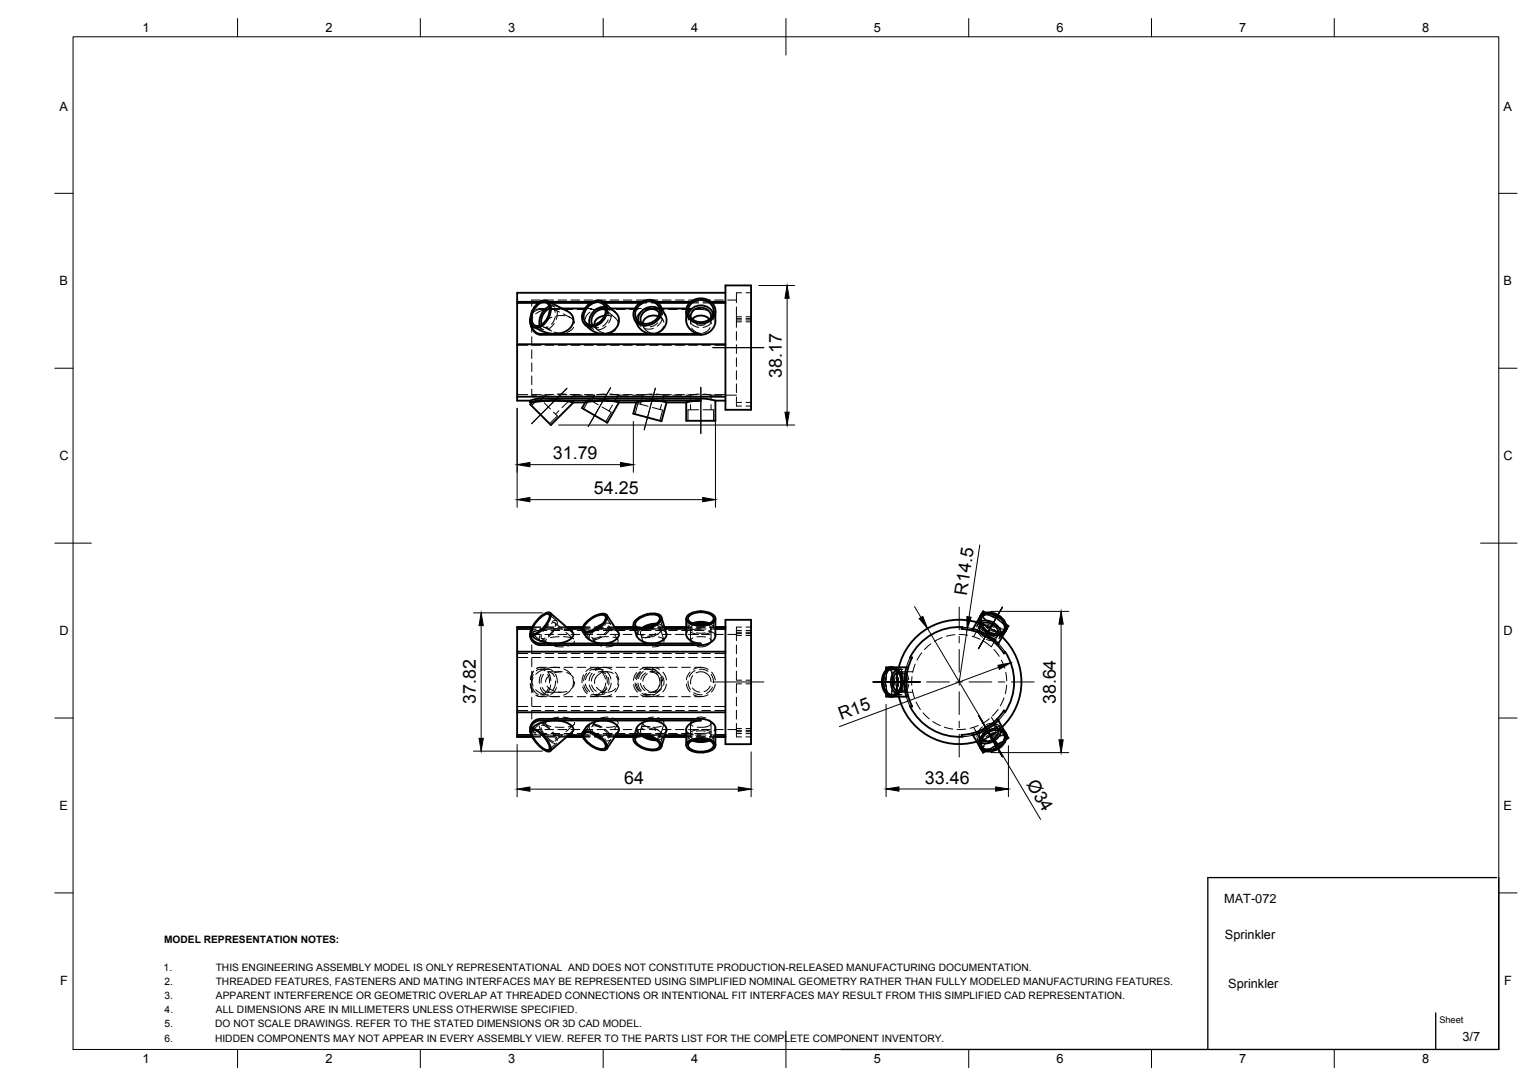
ISO-10303-21;
HEADER;
/* Generated by software containing ST-Developer
 * from STEP Tools, Inc. (www.steptools.com) 
 */

FILE_DESCRIPTION(
/* description */ (''),
/* implementation_level */ '2;1');

FILE_NAME(
/* name */ 'Sprinkler.step',
/* time_stamp */ '2026-10-24T10:30:45-07:00',
/* author */ (''),
/* organization */ (''),
/* preprocessor_version */ 'ST-DEVELOPER v20.2',
/* originating_system */ 'Autodesk Translation Framework v15.15.0.0',
/* authorisation */ '');

FILE_SCHEMA (('AUTOMOTIVE_DESIGN { 1 0 10303 214 3 1 1 }'));
ENDSEC;

DATA;
#10=MECHANICAL_DESIGN_GEOMETRIC_PRESENTATION_REPRESENTATION('',(#77),#5183);
#67=SHAPE_REPRESENTATION_RELATIONSHIP('SRR','None',#5214,#72);
#72=ADVANCED_BREP_SHAPE_REPRESENTATION('',(#82),#5178);
#77=STYLED_ITEM('',(#5247),#82);
#82=MANIFOLD_SOLID_BREP('Sprinkler',#2363);
#87=B_SPLINE_SURFACE_WITH_KNOTS('',3,1,((#4861,#4862),(#4863,#4864),(#4865,
#4866),(#4867,#4868),(#4869,#4870),(#4871,#4872),(#4873,#4874),(#4875,#4876),
(#4877,#4878),(#4879,#4880),(#4881,#4882)),.UNSPECIFIED.,.F.,.F.,.F.,(4,
1,1,1,1,1,1,1,4),(2,2),(3.14159265358979,3.53429173528852,3.92699081698724,
4.31968989868597,4.71238898038469,5.10508806208341,5.49778714378214,5.89048622548086,
6.28318530717959),(0.,0.129347179873149),.UNSPECIFIED.);
#88=B_SPLINE_SURFACE_WITH_KNOTS('',3,1,((#4924,#4925),(#4926,#4927),(#4928,
#4929),(#4930,#4931),(#4932,#4933),(#4934,#4935),(#4936,#4937),(#4938,#4939),
(#4940,#4941),(#4942,#4943),(#4944,#4945)),.UNSPECIFIED.,.F.,.F.,.F.,(4,
1,1,1,1,1,1,1,4),(2,2),(3.14159265358979,3.53429173528851,3.92699081698724,
4.31968989868596,4.71238898038469,5.10508806208341,5.49778714378214,5.89048622548086,
6.28318530717959),(0.,0.129347179873148),.UNSPECIFIED.);
#89=B_SPLINE_SURFACE_WITH_KNOTS('',3,1,((#4987,#4988),(#4989,#4990),(#4991,
#4992),(#4993,#4994),(#4995,#4996),(#4997,#4998),(#4999,#5000),(#5001,#5002),
(#5003,#5004),(#5005,#5006),(#5007,#5008)),.UNSPECIFIED.,.F.,.F.,.F.,(4,
1,1,1,1,1,1,1,4),(2,2),(3.14159265358979,3.53429173528851,3.92699081698723,
4.31968989868596,4.71238898038468,5.10508806208341,5.49778714378213,5.89048622548085,
6.28318530717958),(0.,0.129347179873145),.UNSPECIFIED.);
#90=FACE_BOUND('',#431,.T.);
#91=FACE_BOUND('',#433,.T.);
#92=FACE_BOUND('',#436,.T.);
#93=FACE_BOUND('',#439,.T.);
#94=FACE_BOUND('',#442,.T.);
#95=FACE_BOUND('',#445,.T.);
#96=FACE_BOUND('',#448,.T.);
#97=FACE_BOUND('',#451,.T.);
#98=FACE_BOUND('',#454,.T.);
#99=FACE_BOUND('',#457,.T.);
#100=FACE_BOUND('',#460,.T.);
#101=FACE_BOUND('',#461,.T.);
#102=FACE_BOUND('',#462,.T.);
#103=FACE_BOUND('',#463,.T.);
#104=FACE_BOUND('',#464,.T.);
#105=FACE_BOUND('',#465,.T.);
#106=FACE_BOUND('',#466,.T.);
#107=FACE_BOUND('',#467,.T.);
#108=FACE_BOUND('',#468,.T.);
#109=FACE_BOUND('',#469,.T.);
#110=FACE_BOUND('',#470,.T.);
#111=FACE_BOUND('',#471,.T.);
#112=FACE_BOUND('',#474,.T.);
#113=FACE_BOUND('',#481,.T.);
#114=FACE_BOUND('',#484,.T.);
#115=FACE_BOUND('',#487,.T.);
#116=FACE_BOUND('',#490,.T.);
#117=FACE_BOUND('',#493,.T.);
#118=FACE_BOUND('',#496,.T.);
#119=FACE_BOUND('',#499,.T.);
#120=FACE_BOUND('',#502,.T.);
#121=FACE_BOUND('',#513,.T.);
#122=FACE_BOUND('',#516,.T.);
#123=FACE_BOUND('',#519,.T.);
#124=FACE_BOUND('',#522,.T.);
#125=FACE_BOUND('',#525,.T.);
#126=FACE_BOUND('',#528,.T.);
#127=FACE_BOUND('',#531,.T.);
#128=FACE_BOUND('',#534,.T.);
#129=FACE_BOUND('',#542,.T.);
#130=FACE_BOUND('',#549,.T.);
#131=FACE_BOUND('',#556,.T.);
#144=PLANE('',#2456);
#145=PLANE('',#2461);
#146=PLANE('',#2464);
#147=PLANE('',#2466);
#148=PLANE('',#2470);
#149=PLANE('',#2474);
#150=PLANE('',#2478);
#151=PLANE('',#2482);
#152=PLANE('',#2486);
#153=PLANE('',#2490);
#154=PLANE('',#2494);
#155=PLANE('',#2500);
#156=PLANE('',#2501);
#157=PLANE('',#2509);
#158=PLANE('',#2513);
#159=PLANE('',#2517);
#160=PLANE('',#2521);
#161=PLANE('',#2525);
#162=PLANE('',#2529);
#163=PLANE('',#2533);
#164=PLANE('',#2537);
#165=PLANE('',#2557);
#166=PLANE('',#2560);
#167=PLANE('',#2563);
#168=PLANE('',#2566);
#169=PLANE('',#2569);
#170=PLANE('',#2572);
#171=PLANE('',#2575);
#172=PLANE('',#2578);
#173=PLANE('',#2581);
#174=PLANE('',#2582);
#175=PLANE('',#2583);
#176=PLANE('',#2584);
#177=PLANE('',#2586);
#178=PLANE('',#2587);
#179=PLANE('',#2588);
#180=PLANE('',#2589);
#181=PLANE('',#2591);
#182=PLANE('',#2592);
#183=PLANE('',#2593);
#184=PLANE('',#2594);
#185=PLANE('',#2596);
#186=PLANE('',#2597);
#187=PLANE('',#2598);
#188=PLANE('',#2599);
#189=PLANE('',#2600);
#190=PLANE('',#2601);
#191=PLANE('',#2602);
#192=PLANE('',#2603);
#193=PLANE('',#2604);
#206=B_SPLINE_CURVE_WITH_KNOTS('',3,(#3370,#3371,#3372,#3373,#3374,#3375,
#3376,#3377),.UNSPECIFIED.,.F.,.F.,(4,2,2,4),(0.801601659973552,0.908686694681274,
1.06147652934293,1.21426636400458),.UNSPECIFIED.);
#207=B_SPLINE_CURVE_WITH_KNOTS('',3,(#3379,#3380,#3381,#3382,#3383,#3384,
#3385,#3386,#3387,#3388,#3389,#3390,#3391,#3392),.UNSPECIFIED.,.F.,.F.,
(4,2,2,2,2,2,4),(0.,0.152789834661652,0.305579669323305,0.456356425662796,
0.607133182002287,0.757909938341781,0.801601659973552),.UNSPECIFIED.);
#208=B_SPLINE_CURVE_WITH_KNOTS('',3,(#3396,#3397,#3398,#3399,#3400,#3401,
#3402,#3403,#3404,#3405,#3406,#3407,#3408,#3409,#3410,#3411),
 .UNSPECIFIED.,.F.,.F.,(4,2,2,2,2,2,2,4),(1.41258149283994,1.51470567835646,
1.66615965590029,1.81761363344413,1.96906761098797,2.12052158853181,2.27200321656199,
2.42348484459217),.UNSPECIFIED.);
#209=B_SPLINE_CURVE_WITH_KNOTS('',3,(#3412,#3413,#3414,#3415,#3416,#3417),
 .UNSPECIFIED.,.F.,.F.,(4,2,4),(1.21174242229609,1.36322405032627,1.41258149283994),
 .UNSPECIFIED.);
#210=B_SPLINE_CURVE_WITH_KNOTS('',3,(#3422,#3423,#3424,#3425,#3426,#3427,
#3428,#3429),.UNSPECIFIED.,.F.,.F.,(4,2,2,4),(0.810459053731311,0.931112082660273,
1.09792489409666,1.26473770553305),.UNSPECIFIED.);
#211=B_SPLINE_CURVE_WITH_KNOTS('',3,(#3431,#3432,#3433,#3434,#3435,#3436,
#3437,#3438,#3439,#3440,#3441,#3442,#3443,#3444),.UNSPECIFIED.,.F.,.F.,
(4,2,2,2,2,2,4),(0.,0.166812811436392,0.333625622872784,0.482997237819655,
0.632368852766526,0.781740467713401,0.810459053731311),.UNSPECIFIED.);
#212=B_SPLINE_CURVE_WITH_KNOTS('',3,(#3446,#3447,#3448,#3449,#3450,#3451,
#3452,#3453,#3454,#3455,#3456,#3457,#3458,#3459,#3460,#3461,#3462,#3463),
 .UNSPECIFIED.,.F.,.F.,(4,2,2,2,2,2,2,2,4),(1.21426636400458,1.37281902636882,
1.53137168873306,1.68587949128402,1.84038729383497,1.99489509638593,2.14940289893689,
2.30795556130114,2.46650822366539),.UNSPECIFIED.);
#213=B_SPLINE_CURVE_WITH_KNOTS('',3,(#3468,#3469,#3470,#3471,#3472,#3473,
#3474,#3475,#3476,#3477),.UNSPECIFIED.,.F.,.F.,(4,2,2,2,4),(0.84921255840186,
0.855460999411689,1.0133776521287,1.20423317275903,1.39508869338936),
 .UNSPECIFIED.);
#214=B_SPLINE_CURVE_WITH_KNOTS('',3,(#3479,#3480,#3481,#3482,#3483,#3484,
#3485,#3486,#3487,#3488,#3489,#3490),.UNSPECIFIED.,.F.,.F.,(4,2,2,2,2,4),
(0.,0.19085552063033,0.38171104126066,0.539627693977667,0.697544346694674,
0.84921255840186),.UNSPECIFIED.);
#215=B_SPLINE_CURVE_WITH_KNOTS('',3,(#3492,#3493,#3494,#3495,#3496,#3497,
#3498,#3499,#3500,#3501,#3502,#3503,#3504,#3505,#3506,#3507,#3508,#3509),
 .UNSPECIFIED.,.F.,.F.,(4,2,2,2,2,2,2,2,4),(1.26473770553305,1.44115993597425,
1.61758216641546,1.77878219205947,1.93998221770349,2.10118224334752,2.26238226899155,
2.43880449943275,2.61522672987395),.UNSPECIFIED.);
#216=B_SPLINE_CURVE_WITH_KNOTS('',3,(#3513,#3514,#3515,#3516,#3517,#3518,
#3519,#3520,#3521,#3522,#3523,#3524,#3525,#3526,#3527,#3528,#3529,#3530,
#3531,#3532,#3533,#3534),.UNSPECIFIED.,.F.,.F.,(4,2,2,2,2,2,2,2,2,2,4),
(1.39508869338936,1.63068735474474,1.86628601610013,2.01895939966093,2.09529609144134,
2.17163278322174,2.24796947500215,2.32430616678255,2.47697955034337,2.71257821169876,
2.94817687305416),.UNSPECIFIED.);
#217=B_SPLINE_CURVE_WITH_KNOTS('',3,(#3537,#3538,#3539,#3540,#3541,#3542,
#3543,#3544,#3545,#3546,#3547,#3548,#3549,#3550,#3551,#3552,#3553,#3554,
#3555,#3556,#3557,#3558,#3559,#3560,#3561,#3562),.UNSPECIFIED.,.F.,.F.,
(4,2,2,2,2,2,2,2,2,2,2,2,4),(0.,0.0444658256706816,0.109825747467382,0.210987273969983,
0.363115011869221,0.476603266918211,0.543343022865724,0.610052308554092,
0.7232875236507,0.87579543247345,0.97697424211648,1.04237097445545,1.08685368328188),
 .UNSPECIFIED.);
#218=B_SPLINE_CURVE_WITH_KNOTS('',3,(#3577,#3578,#3579,#3580,#3581,#3582,
#3583,#3584),.UNSPECIFIED.,.F.,.F.,(4,2,2,4),(0.801601659973551,0.908686694681269,
1.06147652934292,1.21426636400457),.UNSPECIFIED.);
#219=B_SPLINE_CURVE_WITH_KNOTS('',3,(#3586,#3587,#3588,#3589,#3590,#3591,
#3592,#3593,#3594,#3595,#3596,#3597,#3598,#3599),.UNSPECIFIED.,.F.,.F.,
(4,2,2,2,2,2,4),(0.,0.152789834661651,0.305579669323302,0.456356425662796,
0.607133182002289,0.757909938341779,0.801601659973551),.UNSPECIFIED.);
#220=B_SPLINE_CURVE_WITH_KNOTS('',3,(#3603,#3604,#3605,#3606,#3607,#3608,
#3609,#3610,#3611,#3612,#3613,#3614,#3615,#3616,#3617,#3618),
 .UNSPECIFIED.,.F.,.F.,(4,2,2,2,2,2,2,4),(1.41258149283993,1.51470567835645,
1.66615965590029,1.81761363344413,1.96906761098797,2.1205215885318,2.27200321656199,
2.42348484459217),.UNSPECIFIED.);
#221=B_SPLINE_CURVE_WITH_KNOTS('',3,(#3619,#3620,#3621,#3622,#3623,#3624),
 .UNSPECIFIED.,.F.,.F.,(4,2,4),(1.21174242229609,1.36322405032627,1.41258149283993),
 .UNSPECIFIED.);
#222=B_SPLINE_CURVE_WITH_KNOTS('',3,(#3629,#3630,#3631,#3632,#3633,#3634,
#3635,#3636),.UNSPECIFIED.,.F.,.F.,(4,2,2,4),(0.810459053731318,0.931112082660271,
1.09792489409666,1.26473770553306),.UNSPECIFIED.);
#223=B_SPLINE_CURVE_WITH_KNOTS('',3,(#3638,#3639,#3640,#3641,#3642,#3643,
#3644,#3645,#3646,#3647,#3648,#3649,#3650,#3651),.UNSPECIFIED.,.F.,.F.,
(4,2,2,2,2,2,4),(0.,0.166812811436393,0.333625622872785,0.482997237819654,
0.632368852766523,0.781740467713397,0.810459053731318),.UNSPECIFIED.);
#224=B_SPLINE_CURVE_WITH_KNOTS('',3,(#3653,#3654,#3655,#3656,#3657,#3658,
#3659,#3660,#3661,#3662,#3663,#3664,#3665,#3666,#3667,#3668,#3669,#3670),
 .UNSPECIFIED.,.F.,.F.,(4,2,2,2,2,2,2,2,4),(1.21426636400457,1.37281902636881,
1.53137168873306,1.68587949128401,1.84038729383497,1.99489509638593,2.14940289893689,
2.30795556130114,2.46650822366538),.UNSPECIFIED.);
#225=B_SPLINE_CURVE_WITH_KNOTS('',3,(#3675,#3676,#3677,#3678,#3679,#3680,
#3681,#3682),.UNSPECIFIED.,.F.,.F.,(4,2,2,4),(0.848478832255458,0.991796836691898,
1.19347267089766,1.39514850510343),.UNSPECIFIED.);
#226=B_SPLINE_CURVE_WITH_KNOTS('',3,(#3684,#3685,#3686,#3687,#3688,#3689,
#3690,#3691,#3692,#3693,#3694,#3695,#3696,#3697),.UNSPECIFIED.,.F.,.F.,
(4,2,2,2,2,2,4),(0.,0.201675834205757,0.403351668411514,0.550462960481608,
0.697574252551703,0.8446855446218,0.848478832255458),.UNSPECIFIED.);
#227=B_SPLINE_CURVE_WITH_KNOTS('',3,(#3699,#3700,#3701,#3702,#3703,#3704,
#3705,#3706,#3707,#3708,#3709,#3710,#3711,#3712,#3713,#3714,#3715,#3716),
 .UNSPECIFIED.,.F.,.F.,(4,2,2,2,2,2,2,2,4),(1.26473770553306,1.44115993597426,
1.61758216641546,1.77878219205948,1.93998221770349,2.10118224334752,2.26238226899154,
2.43880449943275,2.61522672987395),.UNSPECIFIED.);
#228=B_SPLINE_CURVE_WITH_KNOTS('',3,(#3720,#3721,#3722,#3723,#3724,#3725,
#3726,#3727,#3728,#3729,#3730,#3731,#3732,#3733,#3734,#3735,#3736,#3737,
#3738,#3739,#3740,#3741),.UNSPECIFIED.,.F.,.F.,(4,2,2,2,2,2,2,2,2,2,4),
(1.39514850510343,1.60860320712188,1.82205790914033,1.99791237111712,2.08583960210551,
2.17376683309391,2.26169406408231,2.34962129507071,2.5254757570475,2.73893045906596,
2.95238516108442),.UNSPECIFIED.);
#229=B_SPLINE_CURVE_WITH_KNOTS('',3,(#3744,#3745,#3746,#3747,#3748,#3749,
#3750,#3751,#3752,#3753,#3754,#3755,#3756,#3757,#3758,#3759,#3760,#3761,
#3762,#3763,#3764,#3765,#3766,#3767,#3768,#3769),.UNSPECIFIED.,.F.,.F.,
(4,2,2,2,2,2,2,2,2,2,2,2,4),(0.,0.0444658256707017,0.109825747467453,0.210987273970143,
0.363115011869592,0.4766032669186,0.543343022866364,0.610052308555067,0.723287523653244,
0.875795432478097,0.97697424212264,1.04237097446268,1.08685368328966),
 .UNSPECIFIED.);
#230=B_SPLINE_CURVE_WITH_KNOTS('',3,(#3775,#3776,#3777,#3778,#3779,#3780,
#3781,#3782),.UNSPECIFIED.,.F.,.F.,(4,2,2,4),(0.80160165997355,0.908686694681275,
1.06147652934293,1.21426636400458),.UNSPECIFIED.);
#231=B_SPLINE_CURVE_WITH_KNOTS('',3,(#3784,#3785,#3786,#3787,#3788,#3789,
#3790,#3791,#3792,#3793,#3794,#3795,#3796,#3797),.UNSPECIFIED.,.F.,.F.,
(4,2,2,2,2,2,4),(0.,0.152789834661653,0.305579669323305,0.456356425662799,
0.607133182002292,0.757909938341784,0.80160165997355),.UNSPECIFIED.);
#232=B_SPLINE_CURVE_WITH_KNOTS('',3,(#3801,#3802,#3803,#3804,#3805,#3806,
#3807,#3808,#3809,#3810,#3811,#3812,#3813,#3814,#3815,#3816),
 .UNSPECIFIED.,.F.,.F.,(4,2,2,2,2,2,2,4),(1.41258149283993,1.51470567835645,
1.66615965590029,1.81761363344413,1.96906761098797,2.12052158853181,2.27200321656199,
2.42348484459217),.UNSPECIFIED.);
#233=B_SPLINE_CURVE_WITH_KNOTS('',3,(#3817,#3818,#3819,#3820,#3821,#3822),
 .UNSPECIFIED.,.F.,.F.,(4,2,4),(1.21174242229609,1.36322405032627,1.41258149283993),
 .UNSPECIFIED.);
#234=B_SPLINE_CURVE_WITH_KNOTS('',3,(#3827,#3828,#3829,#3830,#3831,#3832,
#3833,#3834),.UNSPECIFIED.,.F.,.F.,(4,2,2,4),(0.810451797988797,0.931104826917751,
1.09791763835414,1.26473044979053),.UNSPECIFIED.);
#235=B_SPLINE_CURVE_WITH_KNOTS('',3,(#3836,#3837,#3838,#3839,#3840,#3841,
#3842,#3843,#3844,#3845,#3846,#3847,#3848,#3849),.UNSPECIFIED.,.F.,.F.,
(4,2,2,2,2,2,4),(0.,0.163827053405726,0.327654106811452,0.48000785191773,
0.632361597024009,0.781733211970881,0.810451797988797),.UNSPECIFIED.);
#236=B_SPLINE_CURVE_WITH_KNOTS('',3,(#3851,#3852,#3853,#3854,#3855,#3856,
#3857,#3858,#3859,#3860,#3861,#3862,#3863,#3864,#3865,#3866,#3867,#3868),
 .UNSPECIFIED.,.F.,.F.,(4,2,2,2,2,2,2,2,4),(1.21426636400458,1.37281902636882,
1.53137168873306,1.68587949128402,1.84038729383497,1.99489509638594,2.1494028989369,
2.30795556130114,2.46650822366539),.UNSPECIFIED.);
#237=B_SPLINE_CURVE_WITH_KNOTS('',3,(#3873,#3874,#3875,#3876,#3877,#3878,
#3879,#3880,#3881,#3882),.UNSPECIFIED.,.F.,.F.,(4,2,2,2,4),(0.849212558401863,
0.855460999411694,1.01337765212871,1.20423317275904,1.39508869338936),
 .UNSPECIFIED.);
#238=B_SPLINE_CURVE_WITH_KNOTS('',3,(#3884,#3885,#3886,#3887,#3888,#3889,
#3890,#3891,#3892,#3893,#3894,#3895),.UNSPECIFIED.,.F.,.F.,(4,2,2,2,2,4),
(0.,0.190855520630331,0.381711041260663,0.539627693977671,0.697544346694678,
0.849212558401863),.UNSPECIFIED.);
#239=B_SPLINE_CURVE_WITH_KNOTS('',3,(#3897,#3898,#3899,#3900,#3901,#3902,
#3903,#3904,#3905,#3906,#3907,#3908,#3909,#3910,#3911,#3912,#3913,#3914),
 .UNSPECIFIED.,.F.,.F.,(4,2,2,2,2,2,2,2,4),(1.26473044979053,1.45047293867533,
1.63621542756013,1.78793284105988,1.93965025455964,2.0913676680594,2.24308508155916,
2.42882757044396,2.61457005932877),.UNSPECIFIED.);
#240=B_SPLINE_CURVE_WITH_KNOTS('',3,(#3918,#3919,#3920,#3921,#3922,#3923,
#3924,#3925,#3926,#3927,#3928,#3929,#3930,#3931,#3932,#3933,#3934,#3935,
#3936,#3937,#3938,#3939),.UNSPECIFIED.,.F.,.F.,(4,2,2,2,2,2,2,2,2,2,4),
(1.39508869338936,1.63068735474475,1.86628601610013,2.01895939966094,2.09529609144135,
2.17163278322175,2.24796947500216,2.32430616678257,2.47697955034339,2.71257821169878,
2.94817687305417),.UNSPECIFIED.);
#241=B_SPLINE_CURVE_WITH_KNOTS('',3,(#3942,#3943,#3944,#3945,#3946,#3947,
#3948,#3949,#3950,#3951,#3952,#3953,#3954,#3955,#3956,#3957,#3958,#3959,
#3960,#3961,#3962,#3963,#3964,#3965,#3966,#3967),.UNSPECIFIED.,.F.,.F.,
(4,2,2,2,2,2,2,2,2,2,2,2,4),(0.,0.0444658256707104,0.109825747467599,0.210987273970278,
0.3631150118696,0.476603266918339,0.54334302286555,0.610052308553677,0.723287523650531,
0.875795432473984,0.97697424211741,1.0423709744566,1.08685368328313),
 .UNSPECIFIED.);
#242=B_SPLINE_CURVE_WITH_KNOTS('',3,(#4068,#4069,#4070,#4071,#4072,#4073,
#4074,#4075,#4076,#4077,#4078,#4079,#4080,#4081,#4082,#4083,#4084,#4085),
 .UNSPECIFIED.,.F.,.F.,(4,2,2,2,2,2,2,2,4),(-2.42440986895006,-2.27286833474306,
-2.12132680053607,-1.9698171011243,-1.81830740171254,-1.66679770230078,
-1.51528800288901,-1.36374646868202,-1.21220493447502),.UNSPECIFIED.);
#243=B_SPLINE_CURVE_WITH_KNOTS('',3,(#4135,#4136,#4137,#4138,#4139,#4140,
#4141,#4142,#4143,#4144,#4145,#4146,#4147,#4148,#4149,#4150,#4151,#4152,
#4153,#4154,#4155),.UNSPECIFIED.,.F.,.F.,(4,2,2,2,3,2,2,2,2,4),(1.63431795680218,
1.63484051213071,1.74655213492763,1.90358589296679,2.06061965100595,2.19559646985844,
2.33057328871092,2.44200600177385,2.55343871483678,2.66004451397958),
 .UNSPECIFIED.);
#244=B_SPLINE_CURVE_WITH_KNOTS('',3,(#4156,#4157,#4158,#4159,#4160,#4161,
#4162,#4163,#4164,#4165,#4166,#4167,#4168,#4169,#4170,#4171,#4172,#4173,
#4174,#4175,#4176,#4177,#4178,#4179),.UNSPECIFIED.,.F.,.F.,(4,2,2,2,2,2,
2,2,2,2,2,4),(2.66004451397958,2.66487142789972,2.77630414096266,2.91128095981515,
3.04625777866764,3.20329153670679,3.36032529474595,3.47203691754285,3.5278927289413,
3.58374854033975,3.63960435173821,3.69493760780813),.UNSPECIFIED.);
#245=B_SPLINE_CURVE_WITH_KNOTS('',3,(#4182,#4183,#4184,#4185,#4186,#4187,
#4188,#4189,#4190,#4191,#4192,#4193,#4194,#4195,#4196,#4197,#4198,#4199,
#4200,#4201,#4202,#4203,#4204),.UNSPECIFIED.,.F.,.F.,(4,2,2,2,3,2,2,2,2,
2,4),(1.63645246149242,1.6458071028209,1.76735674157733,1.91500283165642,
2.06264892173552,2.21065304350676,2.35865716527801,2.45711954510512,2.55558192493224,
2.65404430475936,2.66124396153498),.UNSPECIFIED.);
#246=B_SPLINE_CURVE_WITH_KNOTS('',3,(#4205,#4206,#4207,#4208,#4209,#4210,
#4211,#4212,#4213,#4214,#4215,#4216,#4217,#4218,#4219,#4220,#4221,#4222,
#4223,#4224,#4225,#4226),.UNSPECIFIED.,.F.,.F.,(4,2,2,2,2,2,2,2,2,2,4),
(2.66124396153498,2.75250668458648,2.90051080635773,3.04851492812899,3.19616101820807,
3.34380710828715,3.46535674704357,3.52613156642178,3.58690638579999,3.64768120517821,
3.69910138322794),.UNSPECIFIED.);
#247=B_SPLINE_CURVE_WITH_KNOTS('',3,(#4229,#4230,#4231,#4232,#4233,#4234,
#4235,#4236,#4237,#4238,#4239,#4240,#4241,#4242,#4243,#4244,#4245,#4246,
#4247,#4248,#4249),.UNSPECIFIED.,.F.,.F.,(4,2,2,3,2,2,2,2,2,4),(1.48658026968319,
1.57668032617585,1.70181043495793,1.82694054374001,1.94229840394621,2.0576562641524,
2.16466765320846,2.27167904226452,2.37869043132058,2.39673280800115),
 .UNSPECIFIED.);
#248=B_SPLINE_CURVE_WITH_KNOTS('',3,(#4250,#4251,#4252,#4253,#4254,#4255,
#4256,#4257,#4258,#4259,#4260,#4261,#4262,#4263,#4264,#4265,#4266,#4267,
#4268,#4269),.UNSPECIFIED.,.F.,.F.,(4,2,2,2,2,2,2,2,2,4),(2.39673280800115,
2.48570182037664,2.60105968058284,2.71641754078903,2.84154764957111,2.96667775835319,
3.07591353624385,3.18514931413451,3.29438509202518,3.3135208134232),
 .UNSPECIFIED.);
#249=B_SPLINE_CURVE_WITH_KNOTS('',3,(#4272,#4273,#4274,#4275,#4276,#4277,
#4278,#4279,#4280,#4281,#4282,#4283,#4284,#4285,#4286,#4287,#4288,#4289,
#4290,#4291,#4292),.UNSPECIFIED.,.F.,.F.,(4,2,2,3,2,2,2,2,2,4),(1.48667142164751,
1.57677147814025,1.70190158692234,1.82703169570442,1.94802136665288,2.06901103760135,
2.17041340390623,2.27181577021112,2.37321813651602,2.39644556681379),
 .UNSPECIFIED.);
#250=B_SPLINE_CURVE_WITH_KNOTS('',3,(#4293,#4294,#4295,#4296,#4297,#4298,
#4299,#4300,#4301,#4302,#4303,#4304,#4305,#4306,#4307,#4308,#4309,#4310,
#4311,#4312),.UNSPECIFIED.,.F.,.F.,(4,2,2,2,2,2,2,2,2,4),(2.39644556681379,
2.47462050282091,2.59561017376938,2.71659984471785,2.84172995349992,2.966860062282,
3.07609584017266,3.18533161806333,3.294567395954,3.31370311735193),
 .UNSPECIFIED.);
#251=B_SPLINE_CURVE_WITH_KNOTS('',3,(#4315,#4316,#4317,#4318,#4319,#4320,
#4321,#4322,#4323,#4324,#4325,#4326,#4327,#4328,#4329,#4330,#4331,#4332,
#4333,#4334,#4335),.UNSPECIFIED.,.F.,.F.,(4,2,2,3,2,2,2,2,2,4),(1.42510602309759,
1.50257240162674,1.61295870334865,1.72334500507057,1.83225417045197,1.94116333583337,
2.04500754168813,2.1488517475429,2.25269595339766,2.2848744256183),
 .UNSPECIFIED.);
#252=B_SPLINE_CURVE_WITH_KNOTS('',3,(#4336,#4337,#4338,#4339,#4340,#4341,
#4342,#4343,#4344,#4345,#4346,#4347,#4348,#4349,#4350,#4351,#4352,#4353,
#4354,#4355),.UNSPECIFIED.,.F.,.F.,(4,2,2,2,2,2,2,2,2,4),(2.2848744256183,
2.35654015925242,2.46544932463382,2.57435849001523,2.68474479173714,2.79513109345905,
2.90282767176861,3.01052425007817,3.11822082838774,3.14845102816816),
 .UNSPECIFIED.);
#253=B_SPLINE_CURVE_WITH_KNOTS('',3,(#4358,#4359,#4360,#4361,#4362,#4363,
#4364,#4365,#4366,#4367,#4368,#4369,#4370,#4371,#4372,#4373,#4374,#4375,
#4376,#4377,#4378),.UNSPECIFIED.,.F.,.F.,(4,2,2,3,2,2,2,2,2,4),(1.42506934481542,
1.50220099251643,1.61276096598296,1.72332093944948,1.83050112648501,1.93768131352053,
2.04324956210919,2.14881781069785,2.25438605928651,2.28497277338716),
 .UNSPECIFIED.);
#254=B_SPLINE_CURVE_WITH_KNOTS('',3,(#4379,#4380,#4381,#4382,#4383,#4384,
#4385,#4386,#4387,#4388,#4389,#4390,#4391,#4392,#4393,#4394,#4395,#4396,
#4397,#4398),.UNSPECIFIED.,.F.,.F.,(4,2,2,2,2,2,2,2,2,4),(2.28497277338716,
2.35995430787517,2.46713449491069,2.57431468194622,2.68487465541274,2.79543462887926,
2.90295645465092,3.01047828042258,3.11800010619425,3.1483902842649),
 .UNSPECIFIED.);
#255=B_SPLINE_CURVE_WITH_KNOTS('',3,(#4401,#4402,#4403,#4404,#4405,#4406,
#4407,#4408,#4409,#4410,#4411,#4412,#4413,#4414,#4415,#4416,#4417,#4418,
#4419,#4420),.UNSPECIFIED.,.F.,.F.,(4,2,2,2,2,2,2,2,2,4),(0.140389663816896,
0.211667950083815,0.317493899242379,0.423319848400943,0.529145797559505,
0.634971746718067,0.740805721759974,0.846639696801881,0.952473671843789,
0.987029360618753),.UNSPECIFIED.);
#256=B_SPLINE_CURVE_WITH_KNOTS('',3,(#4421,#4422,#4423,#4424,#4425,#4426,
#4427,#4428,#4429,#4430,#4431,#4432,#4433,#4434,#4435,#4436,#4437,#4438,
#4439,#4440,#4441),.UNSPECIFIED.,.F.,.F.,(4,2,2,2,2,2,2,3,2,4),(0.987029360618753,
1.0583076468857,1.16413359604426,1.26995954520282,1.37578549436138,1.48161144351995,
1.58744541856186,1.69327939360377,1.79911336864567,1.83366905742066),
 .UNSPECIFIED.);
#257=B_SPLINE_CURVE_WITH_KNOTS('',3,(#4444,#4445,#4446,#4447,#4448,#4449,
#4450,#4451,#4452,#4453,#4454,#4455,#4456,#4457,#4458,#4459,#4460,#4461,
#4462,#4463),.UNSPECIFIED.,.F.,.F.,(4,2,2,2,2,2,2,2,2,4),(0.14038966381692,
0.211667950083817,0.317493899242381,0.423319848400946,0.529145797559508,
0.634971746718069,0.740805721759977,0.846639696801884,0.952473671843792,
0.987029360618756),.UNSPECIFIED.);
#258=B_SPLINE_CURVE_WITH_KNOTS('',3,(#4464,#4465,#4466,#4467,#4468,#4469,
#4470,#4471,#4472,#4473,#4474,#4475,#4476,#4477,#4478,#4479,#4480,#4481,
#4482,#4483,#4484),.UNSPECIFIED.,.F.,.F.,(4,2,2,2,2,2,2,3,2,4),(0.987029360618756,
1.0583076468857,1.16413359604426,1.26995954520282,1.37578549436139,1.48161144351995,
1.58744541856186,1.69327939360377,1.79911336864568,1.83366905742069),
 .UNSPECIFIED.);
#259=B_SPLINE_CURVE_WITH_KNOTS('',3,(#4487,#4488,#4489,#4490,#4491,#4492,
#4493,#4494,#4495,#4496,#4497,#4498,#4499,#4500,#4501,#4502,#4503,#4504,
#4505,#4506,#4507),.UNSPECIFIED.,.F.,.F.,(4,2,2,2,3,2,2,2,2,4),(1.63431795680214,
1.63484051213073,1.74655213492764,1.90358589296679,2.06061965100595,2.19559646985844,
2.33057328871092,2.44200600177386,2.5534387148368,2.66004451397959),
 .UNSPECIFIED.);
#260=B_SPLINE_CURVE_WITH_KNOTS('',3,(#4508,#4509,#4510,#4511,#4512,#4513,
#4514,#4515,#4516,#4517,#4518,#4519,#4520,#4521,#4522,#4523,#4524,#4525,
#4526,#4527,#4528,#4529,#4530,#4531),.UNSPECIFIED.,.F.,.F.,(4,2,2,2,2,2,
2,2,2,2,2,4),(2.66004451397959,2.66487142789973,2.77630414096267,2.91128095981515,
3.04625777866764,3.2032915367068,3.36032529474595,3.47203691754286,3.52789272894132,
3.58374854033977,3.63960435173823,3.69493760780809),.UNSPECIFIED.);
#261=B_SPLINE_CURVE_WITH_KNOTS('',3,(#4534,#4535,#4536,#4537,#4538,#4539,
#4540,#4541,#4542,#4543,#4544,#4545,#4546,#4547,#4548,#4549,#4550,#4551,
#4552,#4553,#4554),.UNSPECIFIED.,.F.,.F.,(4,2,2,3,2,2,2,2,2,4),(1.48658026968317,
1.57668032617585,1.70181043495793,1.82694054374001,1.9422984039462,2.0576562641524,
2.16466765320846,2.27167904226452,2.37869043132058,2.39673280800115),
 .UNSPECIFIED.);
#262=B_SPLINE_CURVE_WITH_KNOTS('',3,(#4555,#4556,#4557,#4558,#4559,#4560,
#4561,#4562,#4563,#4564,#4565,#4566,#4567,#4568,#4569,#4570,#4571,#4572,
#4573,#4574),.UNSPECIFIED.,.F.,.F.,(4,2,2,2,2,2,2,2,2,4),(2.39673280800115,
2.48570182037664,2.60105968058283,2.71641754078903,2.84154764957111,2.96667775835319,
3.07591353624386,3.18514931413453,3.29438509202519,3.31352081342317),
 .UNSPECIFIED.);
#263=B_SPLINE_CURVE_WITH_KNOTS('',3,(#4577,#4578,#4579,#4580,#4581,#4582,
#4583,#4584,#4585,#4586,#4587,#4588,#4589,#4590,#4591,#4592,#4593,#4594,
#4595,#4596,#4597),.UNSPECIFIED.,.F.,.F.,(4,2,2,3,2,2,2,2,2,4),(1.42506934481545,
1.50220099251643,1.61276096598296,1.72332093944948,1.83050112648501,1.93768131352053,
2.04324956210919,2.14881781069785,2.25438605928651,2.28497277338716),
 .UNSPECIFIED.);
#264=B_SPLINE_CURVE_WITH_KNOTS('',3,(#4598,#4599,#4600,#4601,#4602,#4603,
#4604,#4605,#4606,#4607,#4608,#4609,#4610,#4611,#4612,#4613,#4614,#4615,
#4616,#4617),.UNSPECIFIED.,.F.,.F.,(4,2,2,2,2,2,2,2,2,4),(2.28497277338716,
2.35995430787516,2.46713449491069,2.57431468194622,2.68487465541274,2.79543462887926,
2.90295645465092,3.01047828042259,3.11800010619425,3.14839028426493),
 .UNSPECIFIED.);
#265=B_SPLINE_CURVE_WITH_KNOTS('',3,(#4620,#4621,#4622,#4623,#4624,#4625,
#4626,#4627,#4628,#4629,#4630,#4631,#4632,#4633,#4634,#4635,#4636,#4637,
#4638,#4639),.UNSPECIFIED.,.F.,.F.,(4,2,2,2,2,2,2,2,2,4),(0.140389663816901,
0.211667950083817,0.31749389924238,0.423319848400942,0.529145797559504,
0.634971746718067,0.740805721759975,0.846639696801883,0.952473671843791,
0.987029360618755),.UNSPECIFIED.);
#266=B_SPLINE_CURVE_WITH_KNOTS('',3,(#4640,#4641,#4642,#4643,#4644,#4645,
#4646,#4647,#4648,#4649,#4650,#4651,#4652,#4653,#4654,#4655,#4656,#4657,
#4658,#4659,#4660),.UNSPECIFIED.,.F.,.F.,(4,2,2,2,2,2,2,3,2,4),(0.987029360618755,
1.0583076468857,1.16413359604426,1.26995954520283,1.37578549436139,1.48161144351995,
1.58744541856186,1.69327939360377,1.79911336864568,1.83366905742067),
 .UNSPECIFIED.);
#267=B_SPLINE_CURVE_WITH_KNOTS('',3,(#4687,#4688,#4689,#4690,#4691,#4692,
#4693,#4694,#4695,#4696,#4697,#4698,#4699,#4700,#4701,#4702,#4703,#4704),
 .UNSPECIFIED.,.F.,.F.,(4,2,2,2,2,2,2,2,4),(-2.42440986895005,-2.27286833474305,
-2.12132680053606,-1.96981710112429,-1.81830740171253,-1.66679770230077,
-1.51528800288901,-1.36374646868202,-1.21220493447502),.UNSPECIFIED.);
#268=B_SPLINE_CURVE_WITH_KNOTS('',3,(#4716,#4717,#4718,#4719,#4720,#4721,
#4722,#4723,#4724,#4725,#4726,#4727,#4728,#4729,#4730,#4731,#4732,#4733),
 .UNSPECIFIED.,.F.,.F.,(4,2,2,2,2,2,2,2,4),(-2.42440986895003,-2.27286833474304,
-2.12132680053605,-1.96981710112428,-1.81830740171252,-1.66679770230076,
-1.515288002889,-1.36374646868201,-1.21220493447502),.UNSPECIFIED.);
#269=B_SPLINE_CURVE_WITH_KNOTS('',3,(#4883,#4884,#4885,#4886,#4887,#4888,
#4889,#4890,#4891,#4892,#4893,#4894,#4895,#4896,#4897,#4898,#4899,#4900,
#4901,#4902,#4903,#4904,#4905,#4906,#4907,#4908,#4909,#4910),
 .UNSPECIFIED.,.F.,.F.,(4,2,2,2,2,2,2,2,2,2,2,2,2,4),(-1.08391055751389,
-1.04041495858034,-0.976127049627852,-0.875975346180159,-0.713802892781725,
-0.606446034139209,-0.5422685089836,-0.478121096415875,-0.370996668444261,
-0.213675448646841,-0.11261366027741,-0.0448303332672381,-0.0212473968071398,
0.),.UNSPECIFIED.);
#270=B_SPLINE_CURVE_WITH_KNOTS('',3,(#4946,#4947,#4948,#4949,#4950,#4951,
#4952,#4953,#4954,#4955,#4956,#4957,#4958,#4959,#4960,#4961,#4962,#4963,
#4964,#4965,#4966,#4967,#4968,#4969,#4970,#4971,#4972,#4973),
 .UNSPECIFIED.,.F.,.F.,(4,2,2,2,2,2,2,2,2,2,2,2,2,4),(-1.08391055750046,
-1.04041495856732,-0.976127049615459,-0.875975346168904,-0.713802892772233,
-0.606446034130957,-0.542268508976211,-0.478121096409307,-0.370996668439296,
-0.213675448644088,-0.112613660276149,-0.0448303332669679,-0.0212473968071859,
0.),.UNSPECIFIED.);
#271=B_SPLINE_CURVE_WITH_KNOTS('',3,(#5009,#5010,#5011,#5012,#5013,#5014,
#5015,#5016,#5017,#5018,#5019,#5020,#5021,#5022,#5023,#5024,#5025,#5026,
#5027,#5028,#5029,#5030,#5031,#5032,#5033,#5034,#5035,#5036),
 .UNSPECIFIED.,.F.,.F.,(4,2,2,2,2,2,2,2,2,2,2,2,2,4),(-1.0839105575165,
-1.04041495858262,-0.976127049629671,-0.8759753461813,-0.713802892781876,
-0.606446034138857,-0.542268508983049,-0.478121096415206,-0.370996668443923,
-0.21367544864674,-0.112613660277534,-0.0448303332674202,-0.021247396807171,
0.),.UNSPECIFIED.);
#272=FACE_OUTER_BOUND('',#412,.T.);
#273=FACE_OUTER_BOUND('',#413,.T.);
#274=FACE_OUTER_BOUND('',#414,.T.);
#275=FACE_OUTER_BOUND('',#415,.T.);
#276=FACE_OUTER_BOUND('',#416,.T.);
#277=FACE_OUTER_BOUND('',#417,.T.);
#278=FACE_OUTER_BOUND('',#418,.T.);
#279=FACE_OUTER_BOUND('',#419,.T.);
#280=FACE_OUTER_BOUND('',#420,.T.);
#281=FACE_OUTER_BOUND('',#421,.T.);
#282=FACE_OUTER_BOUND('',#422,.T.);
#283=FACE_OUTER_BOUND('',#423,.T.);
#284=FACE_OUTER_BOUND('',#424,.T.);
#285=FACE_OUTER_BOUND('',#425,.T.);
#286=FACE_OUTER_BOUND('',#426,.T.);
#287=FACE_OUTER_BOUND('',#427,.T.);
#288=FACE_OUTER_BOUND('',#428,.T.);
#289=FACE_OUTER_BOUND('',#429,.T.);
#290=FACE_OUTER_BOUND('',#430,.T.);
#291=FACE_OUTER_BOUND('',#432,.T.);
#292=FACE_OUTER_BOUND('',#434,.T.);
#293=FACE_OUTER_BOUND('',#435,.T.);
#294=FACE_OUTER_BOUND('',#437,.T.);
#295=FACE_OUTER_BOUND('',#438,.T.);
#296=FACE_OUTER_BOUND('',#440,.T.);
#297=FACE_OUTER_BOUND('',#441,.T.);
#298=FACE_OUTER_BOUND('',#443,.T.);
#299=FACE_OUTER_BOUND('',#444,.T.);
#300=FACE_OUTER_BOUND('',#446,.T.);
#301=FACE_OUTER_BOUND('',#447,.T.);
#302=FACE_OUTER_BOUND('',#449,.T.);
#303=FACE_OUTER_BOUND('',#450,.T.);
#304=FACE_OUTER_BOUND('',#452,.T.);
#305=FACE_OUTER_BOUND('',#453,.T.);
#306=FACE_OUTER_BOUND('',#455,.T.);
#307=FACE_OUTER_BOUND('',#456,.T.);
#308=FACE_OUTER_BOUND('',#458,.T.);
#309=FACE_OUTER_BOUND('',#459,.T.);
#310=FACE_OUTER_BOUND('',#472,.T.);
#311=FACE_OUTER_BOUND('',#473,.T.);
#312=FACE_OUTER_BOUND('',#475,.T.);
#313=FACE_OUTER_BOUND('',#476,.T.);
#314=FACE_OUTER_BOUND('',#477,.T.);
#315=FACE_OUTER_BOUND('',#478,.T.);
#316=FACE_OUTER_BOUND('',#479,.T.);
#317=FACE_OUTER_BOUND('',#480,.T.);
#318=FACE_OUTER_BOUND('',#482,.T.);
#319=FACE_OUTER_BOUND('',#483,.T.);
#320=FACE_OUTER_BOUND('',#485,.T.);
#321=FACE_OUTER_BOUND('',#486,.T.);
#322=FACE_OUTER_BOUND('',#488,.T.);
#323=FACE_OUTER_BOUND('',#489,.T.);
#324=FACE_OUTER_BOUND('',#491,.T.);
#325=FACE_OUTER_BOUND('',#492,.T.);
#326=FACE_OUTER_BOUND('',#494,.T.);
#327=FACE_OUTER_BOUND('',#495,.T.);
#328=FACE_OUTER_BOUND('',#497,.T.);
#329=FACE_OUTER_BOUND('',#498,.T.);
#330=FACE_OUTER_BOUND('',#500,.T.);
#331=FACE_OUTER_BOUND('',#501,.T.);
#332=FACE_OUTER_BOUND('',#503,.T.);
#333=FACE_OUTER_BOUND('',#504,.T.);
#334=FACE_OUTER_BOUND('',#505,.T.);
#335=FACE_OUTER_BOUND('',#506,.T.);
#336=FACE_OUTER_BOUND('',#507,.T.);
#337=FACE_OUTER_BOUND('',#508,.T.);
#338=FACE_OUTER_BOUND('',#509,.T.);
#339=FACE_OUTER_BOUND('',#510,.T.);
#340=FACE_OUTER_BOUND('',#511,.T.);
#341=FACE_OUTER_BOUND('',#512,.T.);
#342=FACE_OUTER_BOUND('',#514,.T.);
#343=FACE_OUTER_BOUND('',#515,.T.);
#344=FACE_OUTER_BOUND('',#517,.T.);
#345=FACE_OUTER_BOUND('',#518,.T.);
#346=FACE_OUTER_BOUND('',#520,.T.);
#347=FACE_OUTER_BOUND('',#521,.T.);
#348=FACE_OUTER_BOUND('',#523,.T.);
#349=FACE_OUTER_BOUND('',#524,.T.);
#350=FACE_OUTER_BOUND('',#526,.T.);
#351=FACE_OUTER_BOUND('',#527,.T.);
#352=FACE_OUTER_BOUND('',#529,.T.);
#353=FACE_OUTER_BOUND('',#530,.T.);
#354=FACE_OUTER_BOUND('',#532,.T.);
#355=FACE_OUTER_BOUND('',#533,.T.);
#356=FACE_OUTER_BOUND('',#535,.T.);
#357=FACE_OUTER_BOUND('',#536,.T.);
#358=FACE_OUTER_BOUND('',#537,.T.);
#359=FACE_OUTER_BOUND('',#538,.T.);
#360=FACE_OUTER_BOUND('',#539,.T.);
#361=FACE_OUTER_BOUND('',#540,.T.);
#362=FACE_OUTER_BOUND('',#541,.T.);
#363=FACE_OUTER_BOUND('',#543,.T.);
#364=FACE_OUTER_BOUND('',#544,.T.);
#365=FACE_OUTER_BOUND('',#545,.T.);
#366=FACE_OUTER_BOUND('',#546,.T.);
#367=FACE_OUTER_BOUND('',#547,.T.);
#368=FACE_OUTER_BOUND('',#548,.T.);
#369=FACE_OUTER_BOUND('',#550,.T.);
#370=FACE_OUTER_BOUND('',#551,.T.);
#371=FACE_OUTER_BOUND('',#552,.T.);
#372=FACE_OUTER_BOUND('',#553,.T.);
#373=FACE_OUTER_BOUND('',#554,.T.);
#374=FACE_OUTER_BOUND('',#555,.T.);
#375=FACE_OUTER_BOUND('',#557,.T.);
#376=FACE_OUTER_BOUND('',#558,.T.);
#377=FACE_OUTER_BOUND('',#559,.T.);
#378=FACE_OUTER_BOUND('',#560,.T.);
#379=FACE_OUTER_BOUND('',#561,.T.);
#380=FACE_OUTER_BOUND('',#562,.T.);
#381=FACE_OUTER_BOUND('',#563,.T.);
#382=FACE_OUTER_BOUND('',#564,.T.);
#383=FACE_OUTER_BOUND('',#565,.T.);
#412=EDGE_LOOP('',(#1524,#1525,#1526,#1527));
#413=EDGE_LOOP('',(#1528,#1529,#1530,#1531));
#414=EDGE_LOOP('',(#1532,#1533,#1534,#1535));
#415=EDGE_LOOP('',(#1536,#1537,#1538,#1539,#1540,#1541));
#416=EDGE_LOOP('',(#1542,#1543,#1544,#1545,#1546));
#417=EDGE_LOOP('',(#1547,#1548,#1549,#1550,#1551));
#418=EDGE_LOOP('',(#1552,#1553,#1554,#1555));
#419=EDGE_LOOP('',(#1556,#1557,#1558,#1559));
#420=EDGE_LOOP('',(#1560,#1561,#1562,#1563,#1564,#1565));
#421=EDGE_LOOP('',(#1566,#1567,#1568,#1569,#1570));
#422=EDGE_LOOP('',(#1571,#1572,#1573,#1574,#1575));
#423=EDGE_LOOP('',(#1576,#1577,#1578,#1579));
#424=EDGE_LOOP('',(#1580,#1581,#1582,#1583,#1584,#1585));
#425=EDGE_LOOP('',(#1586,#1587,#1588,#1589,#1590));
#426=EDGE_LOOP('',(#1591,#1592,#1593,#1594,#1595));
#427=EDGE_LOOP('',(#1596,#1597,#1598,#1599));
#428=EDGE_LOOP('',(#1600,#1601,#1602,#1603));
#429=EDGE_LOOP('',(#1604,#1605,#1606,#1607));
#430=EDGE_LOOP('',(#1608));
#431=EDGE_LOOP('',(#1609,#1610,#1611,#1612,#1613,#1614,#1615,#1616,#1617,
#1618,#1619,#1620));
#432=EDGE_LOOP('',(#1621));
#433=EDGE_LOOP('',(#1622,#1623,#1624,#1625,#1626,#1627,#1628,#1629,#1630,
#1631,#1632,#1633));
#434=EDGE_LOOP('',(#1634,#1635,#1636,#1637));
#435=EDGE_LOOP('',(#1638,#1639,#1640,#1641,#1642,#1643,#1644,#1645,#1646,
#1647,#1648,#1649));
#436=EDGE_LOOP('',(#1650));
#437=EDGE_LOOP('',(#1651,#1652,#1653,#1654,#1655,#1656,#1657,#1658,#1659,
#1660,#1661,#1662));
#438=EDGE_LOOP('',(#1663));
#439=EDGE_LOOP('',(#1664));
#440=EDGE_LOOP('',(#1665,#1666,#1667,#1668,#1669,#1670,#1671,#1672));
#441=EDGE_LOOP('',(#1673));
#442=EDGE_LOOP('',(#1674));
#443=EDGE_LOOP('',(#1675,#1676,#1677,#1678,#1679,#1680));
#444=EDGE_LOOP('',(#1681));
#445=EDGE_LOOP('',(#1682));
#446=EDGE_LOOP('',(#1683,#1684,#1685,#1686,#1687,#1688));
#447=EDGE_LOOP('',(#1689));
#448=EDGE_LOOP('',(#1690));
#449=EDGE_LOOP('',(#1691,#1692,#1693,#1694,#1695,#1696));
#450=EDGE_LOOP('',(#1697));
#451=EDGE_LOOP('',(#1698));
#452=EDGE_LOOP('',(#1699,#1700,#1701,#1702));
#453=EDGE_LOOP('',(#1703));
#454=EDGE_LOOP('',(#1704));
#455=EDGE_LOOP('',(#1705,#1706,#1707,#1708));
#456=EDGE_LOOP('',(#1709));
#457=EDGE_LOOP('',(#1710));
#458=EDGE_LOOP('',(#1711,#1712,#1713,#1714));
#459=EDGE_LOOP('',(#1715,#1716,#1717,#1718));
#460=EDGE_LOOP('',(#1719,#1720));
#461=EDGE_LOOP('',(#1721,#1722));
#462=EDGE_LOOP('',(#1723,#1724));
#463=EDGE_LOOP('',(#1725,#1726));
#464=EDGE_LOOP('',(#1727,#1728));
#465=EDGE_LOOP('',(#1729,#1730));
#466=EDGE_LOOP('',(#1731,#1732));
#467=EDGE_LOOP('',(#1733,#1734));
#468=EDGE_LOOP('',(#1735,#1736));
#469=EDGE_LOOP('',(#1737,#1738));
#470=EDGE_LOOP('',(#1739,#1740));
#471=EDGE_LOOP('',(#1741,#1742));
#472=EDGE_LOOP('',(#1743));
#473=EDGE_LOOP('',(#1744));
#474=EDGE_LOOP('',(#1745));
#475=EDGE_LOOP('',(#1746,#1747,#1748,#1749));
#476=EDGE_LOOP('',(#1750,#1751,#1752,#1753,#1754));
#477=EDGE_LOOP('',(#1755,#1756,#1757,#1758,#1759));
#478=EDGE_LOOP('',(#1760,#1761,#1762,#1763,#1764));
#479=EDGE_LOOP('',(#1765,#1766,#1767,#1768,#1769));
#480=EDGE_LOOP('',(#1770));
#481=EDGE_LOOP('',(#1771));
#482=EDGE_LOOP('',(#1772,#1773,#1774,#1775,#1776,#1777,#1778,#1779));
#483=EDGE_LOOP('',(#1780));
#484=EDGE_LOOP('',(#1781));
#485=EDGE_LOOP('',(#1782,#1783,#1784,#1785,#1786,#1787,#1788,#1789));
#486=EDGE_LOOP('',(#1790));
#487=EDGE_LOOP('',(#1791));
#488=EDGE_LOOP('',(#1792,#1793,#1794,#1795,#1796,#1797));
#489=EDGE_LOOP('',(#1798));
#490=EDGE_LOOP('',(#1799));
#491=EDGE_LOOP('',(#1800,#1801,#1802,#1803,#1804,#1805));
#492=EDGE_LOOP('',(#1806));
#493=EDGE_LOOP('',(#1807));
#494=EDGE_LOOP('',(#1808,#1809,#1810,#1811,#1812,#1813));
#495=EDGE_LOOP('',(#1814));
#496=EDGE_LOOP('',(#1815));
#497=EDGE_LOOP('',(#1816,#1817,#1818,#1819,#1820,#1821));
#498=EDGE_LOOP('',(#1822));
#499=EDGE_LOOP('',(#1823));
#500=EDGE_LOOP('',(#1824,#1825,#1826,#1827,#1828,#1829));
#501=EDGE_LOOP('',(#1830));
#502=EDGE_LOOP('',(#1831));
#503=EDGE_LOOP('',(#1832,#1833,#1834,#1835,#1836,#1837));
#504=EDGE_LOOP('',(#1838,#1839,#1840,#1841,#1842));
#505=EDGE_LOOP('',(#1843,#1844,#1845,#1846,#1847));
#506=EDGE_LOOP('',(#1848,#1849,#1850,#1851,#1852));
#507=EDGE_LOOP('',(#1853,#1854,#1855,#1856,#1857));
#508=EDGE_LOOP('',(#1858,#1859,#1860,#1861,#1862));
#509=EDGE_LOOP('',(#1863,#1864,#1865,#1866,#1867));
#510=EDGE_LOOP('',(#1868,#1869,#1870,#1871,#1872));
#511=EDGE_LOOP('',(#1873,#1874,#1875,#1876,#1877));
#512=EDGE_LOOP('',(#1878));
#513=EDGE_LOOP('',(#1879));
#514=EDGE_LOOP('',(#1880,#1881,#1882,#1883));
#515=EDGE_LOOP('',(#1884));
#516=EDGE_LOOP('',(#1885));
#517=EDGE_LOOP('',(#1886,#1887,#1888,#1889));
#518=EDGE_LOOP('',(#1890));
#519=EDGE_LOOP('',(#1891));
#520=EDGE_LOOP('',(#1892,#1893,#1894,#1895));
#521=EDGE_LOOP('',(#1896));
#522=EDGE_LOOP('',(#1897));
#523=EDGE_LOOP('',(#1898,#1899,#1900,#1901));
#524=EDGE_LOOP('',(#1902));
#525=EDGE_LOOP('',(#1903));
#526=EDGE_LOOP('',(#1904,#1905,#1906,#1907));
#527=EDGE_LOOP('',(#1908));
#528=EDGE_LOOP('',(#1909));
#529=EDGE_LOOP('',(#1910,#1911,#1912,#1913));
#530=EDGE_LOOP('',(#1914));
#531=EDGE_LOOP('',(#1915));
#532=EDGE_LOOP('',(#1916,#1917,#1918,#1919));
#533=EDGE_LOOP('',(#1920));
#534=EDGE_LOOP('',(#1921));
#535=EDGE_LOOP('',(#1922,#1923,#1924,#1925));
#536=EDGE_LOOP('',(#1926,#1927,#1928,#1929));
#537=EDGE_LOOP('',(#1930,#1931,#1932,#1933));
#538=EDGE_LOOP('',(#1934,#1935,#1936,#1937,#1938,#1939,#1940));
#539=EDGE_LOOP('',(#1941,#1942,#1943,#1944,#1945,#1946,#1947));
#540=EDGE_LOOP('',(#1948,#1949,#1950,#1951));
#541=EDGE_LOOP('',(#1952,#1953,#1954,#1955));
#542=EDGE_LOOP('',(#1956,#1957,#1958,#1959));
#543=EDGE_LOOP('',(#1960,#1961,#1962,#1963));
#544=EDGE_LOOP('',(#1964,#1965,#1966,#1967));
#545=EDGE_LOOP('',(#1968,#1969,#1970,#1971,#1972,#1973,#1974));
#546=EDGE_LOOP('',(#1975,#1976,#1977,#1978,#1979,#1980,#1981));
#547=EDGE_LOOP('',(#1982,#1983,#1984,#1985));
#548=EDGE_LOOP('',(#1986,#1987,#1988,#1989));
#549=EDGE_LOOP('',(#1990,#1991,#1992,#1993));
#550=EDGE_LOOP('',(#1994,#1995,#1996,#1997));
#551=EDGE_LOOP('',(#1998,#1999,#2000,#2001));
#552=EDGE_LOOP('',(#2002,#2003,#2004,#2005,#2006,#2007,#2008));
#553=EDGE_LOOP('',(#2009,#2010,#2011,#2012,#2013,#2014,#2015));
#554=EDGE_LOOP('',(#2016,#2017,#2018,#2019));
#555=EDGE_LOOP('',(#2020,#2021,#2022,#2023));
#556=EDGE_LOOP('',(#2024,#2025,#2026,#2027));
#557=EDGE_LOOP('',(#2028,#2029,#2030,#2031));
#558=EDGE_LOOP('',(#2032,#2033,#2034,#2035));
#559=EDGE_LOOP('',(#2036,#2037,#2038,#2039));
#560=EDGE_LOOP('',(#2040,#2041,#2042,#2043));
#561=EDGE_LOOP('',(#2044,#2045,#2046,#2047));
#562=EDGE_LOOP('',(#2048,#2049,#2050,#2051));
#563=EDGE_LOOP('',(#2052,#2053,#2054,#2055));
#564=EDGE_LOOP('',(#2056,#2057,#2058,#2059));
#565=EDGE_LOOP('',(#2060,#2061,#2062,#2063));
#606=CIRCLE('',#2427,15.);
#607=CIRCLE('',#2428,15.);
#608=CIRCLE('',#2430,15.);
#609=CIRCLE('',#2431,15.);
#610=CIRCLE('',#2433,15.);
#611=CIRCLE('',#2434,15.);
#612=CIRCLE('',#2440,15.);
#613=CIRCLE('',#2441,15.);
#614=CIRCLE('',#2451,15.);
#615=CIRCLE('',#2452,15.);
#616=CIRCLE('',#2454,15.);
#617=CIRCLE('',#2455,15.);
#618=CIRCLE('',#2457,17.);
#619=CIRCLE('',#2458,14.5);
#620=CIRCLE('',#2459,14.5);
#621=CIRCLE('',#2460,14.5);
#622=CIRCLE('',#2462,17.);
#623=CIRCLE('',#2465,12.9999999999984);
#624=CIRCLE('',#2467,14.5);
#625=CIRCLE('',#2468,14.5);
#626=CIRCLE('',#2469,14.5);
#627=CIRCLE('',#2471,4.00000000000012);
#628=CIRCLE('',#2472,3.50000000000012);
#629=CIRCLE('',#2475,4.00000000000001);
#630=CIRCLE('',#2476,3.5);
#631=CIRCLE('',#2479,4.00000000000001);
#632=CIRCLE('',#2480,3.49999999999992);
#633=CIRCLE('',#2483,4.);
#634=CIRCLE('',#2484,3.49999999999998);
#635=CIRCLE('',#2487,3.50000000000012);
#636=CIRCLE('',#2488,2.80000000000012);
#637=CIRCLE('',#2491,3.5);
#638=CIRCLE('',#2492,2.79999999999998);
#639=CIRCLE('',#2495,3.49999999999992);
#640=CIRCLE('',#2496,2.79999999999991);
#641=CIRCLE('',#2499,12.9999999999984);
#642=CIRCLE('',#2502,3.49999999999998);
#643=CIRCLE('',#2503,2.79999999999999);
#644=CIRCLE('',#2510,4.00000000000012);
#645=CIRCLE('',#2511,3.50000000000012);
#646=CIRCLE('',#2514,4.00000000000012);
#647=CIRCLE('',#2515,3.50000000000012);
#648=CIRCLE('',#2518,4.00000000000001);
#649=CIRCLE('',#2519,3.5);
#650=CIRCLE('',#2522,4.00000000000001);
#651=CIRCLE('',#2523,3.5);
#652=CIRCLE('',#2526,4.00000000000001);
#653=CIRCLE('',#2527,3.49999999999992);
#654=CIRCLE('',#2530,4.00000000000001);
#655=CIRCLE('',#2531,3.49999999999992);
#656=CIRCLE('',#2534,4.);
#657=CIRCLE('',#2535,3.49999999999998);
#658=CIRCLE('',#2538,4.);
#659=CIRCLE('',#2539,3.49999999999998);
#660=CIRCLE('',#2542,2.80000000000012);
#661=CIRCLE('',#2544,2.80000000000012);
#662=CIRCLE('',#2546,2.79999999999998);
#663=CIRCLE('',#2548,2.79999999999998);
#664=CIRCLE('',#2550,2.79999999999991);
#665=CIRCLE('',#2552,2.79999999999991);
#666=CIRCLE('',#2554,2.79999999999999);
#667=CIRCLE('',#2556,2.79999999999999);
#668=CIRCLE('',#2558,3.50000000000012);
#669=CIRCLE('',#2561,3.50000000000012);
#670=CIRCLE('',#2564,3.5);
#671=CIRCLE('',#2567,3.5);
#672=CIRCLE('',#2570,3.49999999999992);
#673=CIRCLE('',#2573,3.49999999999992);
#674=CIRCLE('',#2576,3.49999999999998);
#675=CIRCLE('',#2579,3.49999999999998);
#704=LINE('',#3341,#854);
#705=LINE('',#3345,#855);
#706=LINE('',#3350,#856);
#707=LINE('',#3354,#857);
#708=LINE('',#3361,#858);
#709=LINE('',#3364,#859);
#710=LINE('',#3368,#860);
#711=LINE('',#3394,#861);
#712=LINE('',#3420,#862);
#713=LINE('',#3445,#863);
#714=LINE('',#3466,#864);
#715=LINE('',#3491,#865);
#716=LINE('',#3512,#866);
#717=LINE('',#3536,#867);
#718=LINE('',#3568,#868);
#719=LINE('',#3571,#869);
#720=LINE('',#3575,#870);
#721=LINE('',#3601,#871);
#722=LINE('',#3627,#872);
#723=LINE('',#3652,#873);
#724=LINE('',#3673,#874);
#725=LINE('',#3698,#875);
#726=LINE('',#3719,#876);
#727=LINE('',#3743,#877);
#728=LINE('',#3773,#878);
#729=LINE('',#3799,#879);
#730=LINE('',#3825,#880);
#731=LINE('',#3850,#881);
#732=LINE('',#3871,#882);
#733=LINE('',#3896,#883);
#734=LINE('',#3917,#884);
#735=LINE('',#3941,#885);
#736=LINE('',#3973,#886);
#737=LINE('',#3976,#887);
#738=LINE('',#3980,#888);
#739=LINE('',#3984,#889);
#740=LINE('',#3990,#890);
#741=LINE('',#3993,#891);
#742=LINE('',#3995,#892);
#743=LINE('',#3998,#893);
#744=LINE('',#4000,#894);
#745=LINE('',#4003,#895);
#746=LINE('',#4008,#896);
#747=LINE('',#4010,#897);
#748=LINE('',#4011,#898);
#749=LINE('',#4013,#899);
#750=LINE('',#4015,#900);
#751=LINE('',#4016,#901);
#752=LINE('',#4018,#902);
#753=LINE('',#4020,#903);
#754=LINE('',#4021,#904);
#755=LINE('',#4023,#905);
#756=LINE('',#4026,#906);
#757=LINE('',#4028,#907);
#758=LINE('',#4029,#908);
#759=LINE('',#4031,#909);
#760=LINE('',#4033,#910);
#761=LINE('',#4034,#911);
#762=LINE('',#4036,#912);
#763=LINE('',#4038,#913);
#764=LINE('',#4039,#914);
#765=LINE('',#4044,#915);
#766=LINE('',#4047,#916);
#767=LINE('',#4049,#917);
#768=LINE('',#4052,#918);
#769=LINE('',#4054,#919);
#770=LINE('',#4057,#920);
#771=LINE('',#4064,#921);
#772=LINE('',#4066,#922);
#773=LINE('',#4086,#923);
#774=LINE('',#4093,#924);
#775=LINE('',#4100,#925);
#776=LINE('',#4107,#926);
#777=LINE('',#4114,#927);
#778=LINE('',#4121,#928);
#779=LINE('',#4128,#929);
#780=LINE('',#4132,#930);
#781=LINE('',#4668,#931);
#782=LINE('',#4670,#932);
#783=LINE('',#4672,#933);
#784=LINE('',#4674,#934);
#785=LINE('',#4676,#935);
#786=LINE('',#4683,#936);
#787=LINE('',#4685,#937);
#788=LINE('',#4705,#938);
#789=LINE('',#4712,#939);
#790=LINE('',#4714,#940);
#791=LINE('',#4734,#941);
#792=LINE('',#4741,#942);
#793=LINE('',#4748,#943);
#794=LINE('',#4755,#944);
#795=LINE('',#4762,#945);
#796=LINE('',#4769,#946);
#797=LINE('',#4776,#947);
#798=LINE('',#4779,#948);
#799=LINE('',#4783,#949);
#800=LINE('',#4787,#950);
#801=LINE('',#4791,#951);
#802=LINE('',#4795,#952);
#803=LINE('',#4799,#953);
#804=LINE('',#4803,#954);
#805=LINE('',#4807,#955);
#806=LINE('',#4813,#956);
#807=LINE('',#4818,#957);
#808=LINE('',#4823,#958);
#809=LINE('',#4828,#959);
#810=LINE('',#4833,#960);
#811=LINE('',#4838,#961);
#812=LINE('',#4843,#962);
#813=LINE('',#4848,#963);
#814=LINE('',#4850,#964);
#815=LINE('',#4852,#965);
#816=LINE('',#4855,#966);
#817=LINE('',#4856,#967);
#818=LINE('',#4859,#968);
#819=LINE('',#4860,#969);
#820=LINE('',#4913,#970);
#821=LINE('',#4915,#971);
#822=LINE('',#4918,#972);
#823=LINE('',#4919,#973);
#824=LINE('',#4922,#974);
#825=LINE('',#4923,#975);
#826=LINE('',#4976,#976);
#827=LINE('',#4978,#977);
#828=LINE('',#4981,#978);
#829=LINE('',#4982,#979);
#830=LINE('',#4985,#980);
#831=LINE('',#4986,#981);
#832=LINE('',#5039,#982);
#833=LINE('',#5041,#983);
#834=LINE('',#5044,#984);
#835=LINE('',#5046,#985);
#836=LINE('',#5049,#986);
#837=LINE('',#5051,#987);
#854=VECTOR('',#2684,3.99999999999999);
#855=VECTOR('',#2687,3.99999999999998);
#856=VECTOR('',#2692,3.99999999999999);
#857=VECTOR('',#2695,3.99999999999996);
#858=VECTOR('',#2702,57.);
#859=VECTOR('',#2705,57.);
#860=VECTOR('',#2708,13.3544586520373);
#861=VECTOR('',#2709,13.3544586520371);
#862=VECTOR('',#2712,13.3319433271509);
#863=VECTOR('',#2713,13.3319433271509);
#864=VECTOR('',#2716,13.2704303156128);
#865=VECTOR('',#2717,13.2704303156126);
#866=VECTOR('',#2720,3.88631345570718);
#867=VECTOR('',#2721,3.88631345570666);
#868=VECTOR('',#2726,57.);
#869=VECTOR('',#2729,57.);
#870=VECTOR('',#2732,13.3544586520373);
#871=VECTOR('',#2733,13.3544586520371);
#872=VECTOR('',#2736,13.3319433271511);
#873=VECTOR('',#2737,13.3319433271509);
#874=VECTOR('',#2740,13.2704303156128);
#875=VECTOR('',#2741,13.2704303156126);
#876=VECTOR('',#2744,3.88631345570709);
#877=VECTOR('',#2745,3.88631345570659);
#878=VECTOR('',#2748,13.3544586520373);
#879=VECTOR('',#2749,13.3544586520371);
#880=VECTOR('',#2752,13.331943327151);
#881=VECTOR('',#2753,13.3319433271509);
#882=VECTOR('',#2756,13.2704303156128);
#883=VECTOR('',#2757,13.2704303156126);
#884=VECTOR('',#2760,3.88631345570711);
#885=VECTOR('',#2761,3.8863134557066);
#886=VECTOR('',#2766,57.);
#887=VECTOR('',#2769,57.);
#888=VECTOR('',#2772,3.99999999999998);
#889=VECTOR('',#2775,3.99999999999998);
#890=VECTOR('',#2782,0.561081020730737);
#891=VECTOR('',#2785,0.561081020730727);
#892=VECTOR('',#2786,0.561081020730758);
#893=VECTOR('',#2789,0.561081020730749);
#894=VECTOR('',#2790,0.561081020730754);
#895=VECTOR('',#2793,0.561081020730736);
#896=VECTOR('',#2798,0.999999999999974);
#897=VECTOR('',#2799,1.00000000000001);
#898=VECTOR('',#2800,0.999999999999884);
#899=VECTOR('',#2801,1.);
#900=VECTOR('',#2802,1.00000000000001);
#901=VECTOR('',#2803,0.999999999999921);
#902=VECTOR('',#2804,0.999999999999996);
#903=VECTOR('',#2805,0.999999999999991);
#904=VECTOR('',#2806,0.99999999999989);
#905=VECTOR('',#2809,17.);
#906=VECTOR('',#2812,0.999999999999894);
#907=VECTOR('',#2813,1.00000000000001);
#908=VECTOR('',#2814,0.999999999999984);
#909=VECTOR('',#2815,0.99999999999989);
#910=VECTOR('',#2816,0.999999999999991);
#911=VECTOR('',#2817,0.999999999999996);
#912=VECTOR('',#2818,0.999999999999925);
#913=VECTOR('',#2819,1.00000000000001);
#914=VECTOR('',#2820,1.00000000000002);
#915=VECTOR('',#2825,0.56108102073074);
#916=VECTOR('',#2828,0.561081020730741);
#917=VECTOR('',#2829,0.561081020730736);
#918=VECTOR('',#2832,0.561081020730754);
#919=VECTOR('',#2833,0.561081020730749);
#920=VECTOR('',#2836,0.561081020730719);
#921=VECTOR('',#2845,4.00000000000012);
#922=VECTOR('',#2846,0.519472430034522);
#923=VECTOR('',#2847,0.519472430034611);
#924=VECTOR('',#2856,4.00000000000001);
#925=VECTOR('',#2865,4.00000000000001);
#926=VECTOR('',#2874,4.);
#927=VECTOR('',#2883,3.50000000000012);
#928=VECTOR('',#2892,3.5);
#929=VECTOR('',#2901,3.49999999999992);
#930=VECTOR('',#2906,12.9999999999984);
#931=VECTOR('',#2917,3.49999999999998);
#932=VECTOR('',#2920,2.80000000000012);
#933=VECTOR('',#2923,2.79999999999998);
#934=VECTOR('',#2926,2.79999999999991);
#935=VECTOR('',#2929,2.79999999999999);
#936=VECTOR('',#2938,4.00000000000012);
#937=VECTOR('',#2939,0.519472430034534);
#938=VECTOR('',#2940,0.519472430034598);
#939=VECTOR('',#2949,4.00000000000012);
#940=VECTOR('',#2950,0.519472430034482);
#941=VECTOR('',#2951,0.519472430034555);
#942=VECTOR('',#2960,4.00000000000001);
#943=VECTOR('',#2969,4.00000000000001);
#944=VECTOR('',#2978,4.00000000000001);
#945=VECTOR('',#2987,4.00000000000001);
#946=VECTOR('',#2996,4.);
#947=VECTOR('',#3005,4.);
#948=VECTOR('',#3008,2.80000000000012);
#949=VECTOR('',#3013,2.80000000000012);
#950=VECTOR('',#3018,2.79999999999998);
#951=VECTOR('',#3023,2.79999999999998);
#952=VECTOR('',#3028,2.79999999999991);
#953=VECTOR('',#3033,2.79999999999991);
#954=VECTOR('',#3038,2.79999999999999);
#955=VECTOR('',#3043,2.79999999999999);
#956=VECTOR('',#3052,3.50000000000012);
#957=VECTOR('',#3059,3.50000000000012);
#958=VECTOR('',#3066,3.5);
#959=VECTOR('',#3073,3.5);
#960=VECTOR('',#3080,3.49999999999992);
#961=VECTOR('',#3087,3.49999999999992);
#962=VECTOR('',#3094,3.49999999999998);
#963=VECTOR('',#3101,3.49999999999998);
#964=VECTOR('',#3104,57.);
#965=VECTOR('',#3107,57.);
#966=VECTOR('',#3110,0.519472430034682);
#967=VECTOR('',#3111,43.8431457505075);
#968=VECTOR('',#3114,43.8431457505077);
#969=VECTOR('',#3115,0.519472430034611);
#970=VECTOR('',#3120,57.);
#971=VECTOR('',#3123,57.);
#972=VECTOR('',#3126,0.51947243003468);
#973=VECTOR('',#3127,43.8431457505077);
#974=VECTOR('',#3130,43.8431457505077);
#975=VECTOR('',#3131,0.519472430034606);
#976=VECTOR('',#3136,57.);
#977=VECTOR('',#3139,57.);
#978=VECTOR('',#3142,0.5194724300347);
#979=VECTOR('',#3143,43.8431457505077);
#980=VECTOR('',#3146,43.8431457505077);
#981=VECTOR('',#3147,0.519472430034622);
#982=VECTOR('',#3152,3.99999999999998);
#983=VECTOR('',#3155,3.99999999999998);
#984=VECTOR('',#3160,3.99999999999997);
#985=VECTOR('',#3163,4.);
#986=VECTOR('',#3168,3.99999999999998);
#987=VECTOR('',#3171,3.99999999999998);
#1004=VERTEX_POINT('',#3339);
#1005=VERTEX_POINT('',#3340);
#1006=VERTEX_POINT('',#3342);
#1007=VERTEX_POINT('',#3344);
#1008=VERTEX_POINT('',#3348);
#1009=VERTEX_POINT('',#3349);
#1010=VERTEX_POINT('',#3351);
#1011=VERTEX_POINT('',#3353);
#1012=VERTEX_POINT('',#3357);
#1013=VERTEX_POINT('',#3358);
#1014=VERTEX_POINT('',#3360);
#1015=VERTEX_POINT('',#3362);
#1016=VERTEX_POINT('',#3366);
#1017=VERTEX_POINT('',#3367);
#1018=VERTEX_POINT('',#3369);
#1019=VERTEX_POINT('',#3378);
#1020=VERTEX_POINT('',#3393);
#1021=VERTEX_POINT('',#3395);
#1022=VERTEX_POINT('',#3419);
#1023=VERTEX_POINT('',#3421);
#1024=VERTEX_POINT('',#3430);
#1025=VERTEX_POINT('',#3465);
#1026=VERTEX_POINT('',#3467);
#1027=VERTEX_POINT('',#3478);
#1028=VERTEX_POINT('',#3511);
#1029=VERTEX_POINT('',#3535);
#1030=VERTEX_POINT('',#3564);
#1031=VERTEX_POINT('',#3565);
#1032=VERTEX_POINT('',#3567);
#1033=VERTEX_POINT('',#3569);
#1034=VERTEX_POINT('',#3573);
#1035=VERTEX_POINT('',#3574);
#1036=VERTEX_POINT('',#3576);
#1037=VERTEX_POINT('',#3585);
#1038=VERTEX_POINT('',#3600);
#1039=VERTEX_POINT('',#3602);
#1040=VERTEX_POINT('',#3626);
#1041=VERTEX_POINT('',#3628);
#1042=VERTEX_POINT('',#3637);
#1043=VERTEX_POINT('',#3672);
#1044=VERTEX_POINT('',#3674);
#1045=VERTEX_POINT('',#3683);
#1046=VERTEX_POINT('',#3718);
#1047=VERTEX_POINT('',#3742);
#1048=VERTEX_POINT('',#3771);
#1049=VERTEX_POINT('',#3772);
#1050=VERTEX_POINT('',#3774);
#1051=VERTEX_POINT('',#3783);
#1052=VERTEX_POINT('',#3798);
#1053=VERTEX_POINT('',#3800);
#1054=VERTEX_POINT('',#3824);
#1055=VERTEX_POINT('',#3826);
#1056=VERTEX_POINT('',#3835);
#1057=VERTEX_POINT('',#3870);
#1058=VERTEX_POINT('',#3872);
#1059=VERTEX_POINT('',#3883);
#1060=VERTEX_POINT('',#3916);
#1061=VERTEX_POINT('',#3940);
#1062=VERTEX_POINT('',#3969);
#1063=VERTEX_POINT('',#3970);
#1064=VERTEX_POINT('',#3972);
#1065=VERTEX_POINT('',#3974);
#1066=VERTEX_POINT('',#3978);
#1067=VERTEX_POINT('',#3979);
#1068=VERTEX_POINT('',#3981);
#1069=VERTEX_POINT('',#3983);
#1070=VERTEX_POINT('',#3987);
#1071=VERTEX_POINT('',#3989);
#1072=VERTEX_POINT('',#3991);
#1073=VERTEX_POINT('',#3994);
#1074=VERTEX_POINT('',#3996);
#1075=VERTEX_POINT('',#3999);
#1076=VERTEX_POINT('',#4001);
#1077=VERTEX_POINT('',#4005);
#1078=VERTEX_POINT('',#4007);
#1079=VERTEX_POINT('',#4009);
#1080=VERTEX_POINT('',#4012);
#1081=VERTEX_POINT('',#4014);
#1082=VERTEX_POINT('',#4017);
#1083=VERTEX_POINT('',#4019);
#1084=VERTEX_POINT('',#4025);
#1085=VERTEX_POINT('',#4027);
#1086=VERTEX_POINT('',#4030);
#1087=VERTEX_POINT('',#4032);
#1088=VERTEX_POINT('',#4035);
#1089=VERTEX_POINT('',#4037);
#1090=VERTEX_POINT('',#4040);
#1091=VERTEX_POINT('',#4043);
#1092=VERTEX_POINT('',#4045);
#1093=VERTEX_POINT('',#4048);
#1094=VERTEX_POINT('',#4050);
#1095=VERTEX_POINT('',#4053);
#1096=VERTEX_POINT('',#4055);
#1097=VERTEX_POINT('',#4059);
#1098=VERTEX_POINT('',#4061);
#1099=VERTEX_POINT('',#4065);
#1100=VERTEX_POINT('',#4067);
#1101=VERTEX_POINT('',#4088);
#1102=VERTEX_POINT('',#4090);
#1103=VERTEX_POINT('',#4095);
#1104=VERTEX_POINT('',#4097);
#1105=VERTEX_POINT('',#4102);
#1106=VERTEX_POINT('',#4104);
#1107=VERTEX_POINT('',#4109);
#1108=VERTEX_POINT('',#4111);
#1109=VERTEX_POINT('',#4116);
#1110=VERTEX_POINT('',#4118);
#1111=VERTEX_POINT('',#4123);
#1112=VERTEX_POINT('',#4125);
#1113=VERTEX_POINT('',#4130);
#1114=VERTEX_POINT('',#4133);
#1115=VERTEX_POINT('',#4134);
#1116=VERTEX_POINT('',#4180);
#1117=VERTEX_POINT('',#4181);
#1118=VERTEX_POINT('',#4227);
#1119=VERTEX_POINT('',#4228);
#1120=VERTEX_POINT('',#4270);
#1121=VERTEX_POINT('',#4271);
#1122=VERTEX_POINT('',#4313);
#1123=VERTEX_POINT('',#4314);
#1124=VERTEX_POINT('',#4356);
#1125=VERTEX_POINT('',#4357);
#1126=VERTEX_POINT('',#4399);
#1127=VERTEX_POINT('',#4400);
#1128=VERTEX_POINT('',#4442);
#1129=VERTEX_POINT('',#4443);
#1130=VERTEX_POINT('',#4485);
#1131=VERTEX_POINT('',#4486);
#1132=VERTEX_POINT('',#4532);
#1133=VERTEX_POINT('',#4533);
#1134=VERTEX_POINT('',#4575);
#1135=VERTEX_POINT('',#4576);
#1136=VERTEX_POINT('',#4618);
#1137=VERTEX_POINT('',#4619);
#1138=VERTEX_POINT('',#4663);
#1139=VERTEX_POINT('',#4665);
#1140=VERTEX_POINT('',#4678);
#1141=VERTEX_POINT('',#4680);
#1142=VERTEX_POINT('',#4684);
#1143=VERTEX_POINT('',#4686);
#1144=VERTEX_POINT('',#4707);
#1145=VERTEX_POINT('',#4709);
#1146=VERTEX_POINT('',#4713);
#1147=VERTEX_POINT('',#4715);
#1148=VERTEX_POINT('',#4736);
#1149=VERTEX_POINT('',#4738);
#1150=VERTEX_POINT('',#4743);
#1151=VERTEX_POINT('',#4745);
#1152=VERTEX_POINT('',#4750);
#1153=VERTEX_POINT('',#4752);
#1154=VERTEX_POINT('',#4757);
#1155=VERTEX_POINT('',#4759);
#1156=VERTEX_POINT('',#4764);
#1157=VERTEX_POINT('',#4766);
#1158=VERTEX_POINT('',#4771);
#1159=VERTEX_POINT('',#4773);
#1160=VERTEX_POINT('',#4778);
#1161=VERTEX_POINT('',#4782);
#1162=VERTEX_POINT('',#4786);
#1163=VERTEX_POINT('',#4790);
#1164=VERTEX_POINT('',#4794);
#1165=VERTEX_POINT('',#4798);
#1166=VERTEX_POINT('',#4802);
#1167=VERTEX_POINT('',#4806);
#1168=VERTEX_POINT('',#4810);
#1169=VERTEX_POINT('',#4815);
#1170=VERTEX_POINT('',#4820);
#1171=VERTEX_POINT('',#4825);
#1172=VERTEX_POINT('',#4830);
#1173=VERTEX_POINT('',#4835);
#1174=VERTEX_POINT('',#4840);
#1175=VERTEX_POINT('',#4845);
#1176=VERTEX_POINT('',#4854);
#1177=VERTEX_POINT('',#4858);
#1178=VERTEX_POINT('',#4917);
#1179=VERTEX_POINT('',#4921);
#1180=VERTEX_POINT('',#4980);
#1181=VERTEX_POINT('',#4984);
#1210=EDGE_CURVE('',#1004,#1005,#704,.F.);
#1211=EDGE_CURVE('',#1006,#1004,#606,.T.);
#1212=EDGE_CURVE('',#1007,#1006,#705,.T.);
#1213=EDGE_CURVE('',#1007,#1005,#607,.T.);
#1214=EDGE_CURVE('',#1008,#1009,#706,.T.);
#1215=EDGE_CURVE('',#1008,#1010,#608,.T.);
#1216=EDGE_CURVE('',#1011,#1010,#707,.F.);
#1217=EDGE_CURVE('',#1009,#1011,#609,.T.);
#1218=EDGE_CURVE('',#1012,#1013,#610,.T.);
#1219=EDGE_CURVE('',#1013,#1014,#708,.F.);
#1220=EDGE_CURVE('',#1015,#1014,#611,.T.);
#1221=EDGE_CURVE('',#1015,#1012,#709,.T.);
#1222=EDGE_CURVE('',#1016,#1017,#710,.T.);
#1223=EDGE_CURVE('',#1018,#1016,#206,.T.);
#1224=EDGE_CURVE('',#1019,#1018,#207,.T.);
#1225=EDGE_CURVE('',#1020,#1019,#711,.F.);
#1226=EDGE_CURVE('',#1021,#1020,#208,.T.);
#1227=EDGE_CURVE('',#1017,#1021,#209,.T.);
#1228=EDGE_CURVE('',#1022,#1016,#712,.T.);
#1229=EDGE_CURVE('',#1023,#1022,#210,.T.);
#1230=EDGE_CURVE('',#1024,#1023,#211,.T.);
#1231=EDGE_CURVE('',#1019,#1024,#713,.F.);
#1232=EDGE_CURVE('',#1016,#1019,#212,.T.);
#1233=EDGE_CURVE('',#1025,#1022,#714,.T.);
#1234=EDGE_CURVE('',#1026,#1025,#213,.T.);
#1235=EDGE_CURVE('',#1027,#1026,#214,.T.);
#1236=EDGE_CURVE('',#1024,#1027,#715,.F.);
#1237=EDGE_CURVE('',#1022,#1024,#215,.T.);
#1238=EDGE_CURVE('',#1027,#1028,#716,.F.);
#1239=EDGE_CURVE('',#1025,#1027,#216,.T.);
#1240=EDGE_CURVE('',#1029,#1025,#717,.T.);
#1241=EDGE_CURVE('',#1028,#1029,#217,.T.);
#1242=EDGE_CURVE('',#1030,#1031,#612,.T.);
#1243=EDGE_CURVE('',#1031,#1032,#718,.F.);
#1244=EDGE_CURVE('',#1033,#1032,#613,.T.);
#1245=EDGE_CURVE('',#1033,#1030,#719,.T.);
#1246=EDGE_CURVE('',#1034,#1035,#720,.T.);
#1247=EDGE_CURVE('',#1036,#1034,#218,.T.);
#1248=EDGE_CURVE('',#1037,#1036,#219,.T.);
#1249=EDGE_CURVE('',#1038,#1037,#721,.F.);
#1250=EDGE_CURVE('',#1039,#1038,#220,.T.);
#1251=EDGE_CURVE('',#1035,#1039,#221,.T.);
#1252=EDGE_CURVE('',#1040,#1034,#722,.T.);
#1253=EDGE_CURVE('',#1041,#1040,#222,.T.);
#1254=EDGE_CURVE('',#1042,#1041,#223,.T.);
#1255=EDGE_CURVE('',#1037,#1042,#723,.F.);
#1256=EDGE_CURVE('',#1034,#1037,#224,.T.);
#1257=EDGE_CURVE('',#1043,#1040,#724,.T.);
#1258=EDGE_CURVE('',#1044,#1043,#225,.T.);
#1259=EDGE_CURVE('',#1045,#1044,#226,.T.);
#1260=EDGE_CURVE('',#1042,#1045,#725,.F.);
#1261=EDGE_CURVE('',#1040,#1042,#227,.T.);
#1262=EDGE_CURVE('',#1045,#1046,#726,.F.);
#1263=EDGE_CURVE('',#1043,#1045,#228,.T.);
#1264=EDGE_CURVE('',#1047,#1043,#727,.T.);
#1265=EDGE_CURVE('',#1046,#1047,#229,.T.);
#1266=EDGE_CURVE('',#1048,#1049,#728,.T.);
#1267=EDGE_CURVE('',#1050,#1048,#230,.T.);
#1268=EDGE_CURVE('',#1051,#1050,#231,.T.);
#1269=EDGE_CURVE('',#1052,#1051,#729,.F.);
#1270=EDGE_CURVE('',#1053,#1052,#232,.T.);
#1271=EDGE_CURVE('',#1049,#1053,#233,.T.);
#1272=EDGE_CURVE('',#1054,#1048,#730,.T.);
#1273=EDGE_CURVE('',#1055,#1054,#234,.T.);
#1274=EDGE_CURVE('',#1056,#1055,#235,.T.);
#1275=EDGE_CURVE('',#1051,#1056,#731,.F.);
#1276=EDGE_CURVE('',#1048,#1051,#236,.T.);
#1277=EDGE_CURVE('',#1057,#1054,#732,.T.);
#1278=EDGE_CURVE('',#1058,#1057,#237,.T.);
#1279=EDGE_CURVE('',#1059,#1058,#238,.T.);
#1280=EDGE_CURVE('',#1056,#1059,#733,.F.);
#1281=EDGE_CURVE('',#1054,#1056,#239,.T.);
#1282=EDGE_CURVE('',#1059,#1060,#734,.F.);
#1283=EDGE_CURVE('',#1057,#1059,#240,.T.);
#1284=EDGE_CURVE('',#1061,#1057,#735,.T.);
#1285=EDGE_CURVE('',#1060,#1061,#241,.T.);
#1286=EDGE_CURVE('',#1062,#1063,#614,.T.);
#1287=EDGE_CURVE('',#1062,#1064,#736,.T.);
#1288=EDGE_CURVE('',#1064,#1065,#615,.T.);
#1289=EDGE_CURVE('',#1065,#1063,#737,.F.);
#1290=EDGE_CURVE('',#1066,#1067,#738,.T.);
#1291=EDGE_CURVE('',#1066,#1068,#616,.T.);
#1292=EDGE_CURVE('',#1069,#1068,#739,.F.);
#1293=EDGE_CURVE('',#1067,#1069,#617,.T.);
#1294=EDGE_CURVE('',#1070,#1070,#618,.T.);
#1295=EDGE_CURVE('',#1071,#1064,#740,.T.);
#1296=EDGE_CURVE('',#1072,#1071,#619,.F.);
#1297=EDGE_CURVE('',#1072,#1013,#741,.T.);
#1298=EDGE_CURVE('',#1073,#1012,#742,.T.);
#1299=EDGE_CURVE('',#1074,#1073,#620,.F.);
#1300=EDGE_CURVE('',#1074,#1031,#743,.T.);
#1301=EDGE_CURVE('',#1075,#1030,#744,.T.);
#1302=EDGE_CURVE('',#1076,#1075,#621,.F.);
#1303=EDGE_CURVE('',#1076,#1065,#745,.T.);
#1304=EDGE_CURVE('',#1077,#1077,#622,.T.);
#1305=EDGE_CURVE('',#1078,#1004,#746,.T.);
#1306=EDGE_CURVE('',#1079,#1078,#747,.T.);
#1307=EDGE_CURVE('',#1009,#1079,#748,.T.);
#1308=EDGE_CURVE('',#1080,#1011,#749,.T.);
#1309=EDGE_CURVE('',#1081,#1080,#750,.T.);
#1310=EDGE_CURVE('',#1067,#1081,#751,.T.);
#1311=EDGE_CURVE('',#1082,#1069,#752,.T.);
#1312=EDGE_CURVE('',#1083,#1082,#753,.T.);
#1313=EDGE_CURVE('',#1006,#1083,#754,.T.);
#1314=EDGE_CURVE('',#1077,#1070,#755,.T.);
#1315=EDGE_CURVE('',#1008,#1084,#756,.T.);
#1316=EDGE_CURVE('',#1084,#1085,#757,.T.);
#1317=EDGE_CURVE('',#1085,#1005,#758,.T.);
#1318=EDGE_CURVE('',#1007,#1086,#759,.T.);
#1319=EDGE_CURVE('',#1086,#1087,#760,.T.);
#1320=EDGE_CURVE('',#1087,#1068,#761,.T.);
#1321=EDGE_CURVE('',#1066,#1088,#762,.T.);
#1322=EDGE_CURVE('',#1088,#1089,#763,.T.);
#1323=EDGE_CURVE('',#1089,#1010,#764,.T.);
#1324=EDGE_CURVE('',#1090,#1090,#623,.T.);
#1325=EDGE_CURVE('',#1091,#1014,#765,.T.);
#1326=EDGE_CURVE('',#1092,#1091,#624,.F.);
#1327=EDGE_CURVE('',#1062,#1092,#766,.T.);
#1328=EDGE_CURVE('',#1093,#1063,#767,.T.);
#1329=EDGE_CURVE('',#1094,#1093,#625,.F.);
#1330=EDGE_CURVE('',#1033,#1094,#768,.T.);
#1331=EDGE_CURVE('',#1095,#1032,#769,.T.);
#1332=EDGE_CURVE('',#1096,#1095,#626,.F.);
#1333=EDGE_CURVE('',#1015,#1096,#770,.T.);
#1334=EDGE_CURVE('',#1097,#1097,#627,.T.);
#1335=EDGE_CURVE('',#1098,#1098,#628,.T.);
#1336=EDGE_CURVE('',#1097,#1053,#771,.T.);
#1337=EDGE_CURVE('',#1099,#1052,#772,.T.);
#1338=EDGE_CURVE('',#1099,#1100,#242,.T.);
#1339=EDGE_CURVE('',#1100,#1049,#773,.T.);
#1340=EDGE_CURVE('',#1101,#1101,#629,.T.);
#1341=EDGE_CURVE('',#1102,#1102,#630,.T.);
#1342=EDGE_CURVE('',#1101,#1050,#774,.T.);
#1343=EDGE_CURVE('',#1103,#1103,#631,.T.);
#1344=EDGE_CURVE('',#1104,#1104,#632,.T.);
#1345=EDGE_CURVE('',#1103,#1055,#775,.T.);
#1346=EDGE_CURVE('',#1105,#1105,#633,.T.);
#1347=EDGE_CURVE('',#1106,#1106,#634,.T.);
#1348=EDGE_CURVE('',#1105,#1058,#776,.T.);
#1349=EDGE_CURVE('',#1107,#1107,#635,.T.);
#1350=EDGE_CURVE('',#1108,#1108,#636,.T.);
#1351=EDGE_CURVE('',#1107,#1098,#777,.T.);
#1352=EDGE_CURVE('',#1109,#1109,#637,.T.);
#1353=EDGE_CURVE('',#1110,#1110,#638,.T.);
#1354=EDGE_CURVE('',#1109,#1102,#778,.T.);
#1355=EDGE_CURVE('',#1111,#1111,#639,.T.);
#1356=EDGE_CURVE('',#1112,#1112,#640,.T.);
#1357=EDGE_CURVE('',#1111,#1104,#779,.T.);
#1358=EDGE_CURVE('',#1113,#1113,#641,.F.);
#1359=EDGE_CURVE('',#1113,#1090,#780,.T.);
#1360=EDGE_CURVE('',#1114,#1115,#243,.T.);
#1361=EDGE_CURVE('',#1115,#1114,#244,.T.);
#1362=EDGE_CURVE('',#1116,#1117,#245,.T.);
#1363=EDGE_CURVE('',#1117,#1116,#246,.T.);
#1364=EDGE_CURVE('',#1118,#1119,#247,.T.);
#1365=EDGE_CURVE('',#1119,#1118,#248,.T.);
#1366=EDGE_CURVE('',#1120,#1121,#249,.T.);
#1367=EDGE_CURVE('',#1121,#1120,#250,.T.);
#1368=EDGE_CURVE('',#1122,#1123,#251,.T.);
#1369=EDGE_CURVE('',#1123,#1122,#252,.T.);
#1370=EDGE_CURVE('',#1124,#1125,#253,.T.);
#1371=EDGE_CURVE('',#1125,#1124,#254,.T.);
#1372=EDGE_CURVE('',#1126,#1127,#255,.T.);
#1373=EDGE_CURVE('',#1127,#1126,#256,.T.);
#1374=EDGE_CURVE('',#1128,#1129,#257,.T.);
#1375=EDGE_CURVE('',#1129,#1128,#258,.T.);
#1376=EDGE_CURVE('',#1130,#1131,#259,.T.);
#1377=EDGE_CURVE('',#1131,#1130,#260,.T.);
#1378=EDGE_CURVE('',#1132,#1133,#261,.T.);
#1379=EDGE_CURVE('',#1133,#1132,#262,.T.);
#1380=EDGE_CURVE('',#1134,#1135,#263,.T.);
#1381=EDGE_CURVE('',#1135,#1134,#264,.T.);
#1382=EDGE_CURVE('',#1136,#1137,#265,.T.);
#1383=EDGE_CURVE('',#1137,#1136,#266,.T.);
#1384=EDGE_CURVE('',#1138,#1138,#642,.T.);
#1385=EDGE_CURVE('',#1139,#1139,#643,.T.);
#1386=EDGE_CURVE('',#1138,#1106,#781,.T.);
#1387=EDGE_CURVE('',#1137,#1108,#782,.T.);
#1388=EDGE_CURVE('',#1135,#1110,#783,.T.);
#1389=EDGE_CURVE('',#1133,#1112,#784,.T.);
#1390=EDGE_CURVE('',#1131,#1139,#785,.T.);
#1391=EDGE_CURVE('',#1140,#1140,#644,.T.);
#1392=EDGE_CURVE('',#1141,#1141,#645,.T.);
#1393=EDGE_CURVE('',#1140,#1021,#786,.T.);
#1394=EDGE_CURVE('',#1142,#1020,#787,.T.);
#1395=EDGE_CURVE('',#1142,#1143,#267,.T.);
#1396=EDGE_CURVE('',#1143,#1017,#788,.T.);
#1397=EDGE_CURVE('',#1144,#1144,#646,.T.);
#1398=EDGE_CURVE('',#1145,#1145,#647,.T.);
#1399=EDGE_CURVE('',#1144,#1039,#789,.T.);
#1400=EDGE_CURVE('',#1146,#1038,#790,.T.);
#1401=EDGE_CURVE('',#1146,#1147,#268,.T.);
#1402=EDGE_CURVE('',#1147,#1035,#791,.T.);
#1403=EDGE_CURVE('',#1148,#1148,#648,.T.);
#1404=EDGE_CURVE('',#1149,#1149,#649,.T.);
#1405=EDGE_CURVE('',#1148,#1018,#792,.T.);
#1406=EDGE_CURVE('',#1150,#1150,#650,.T.);
#1407=EDGE_CURVE('',#1151,#1151,#651,.T.);
#1408=EDGE_CURVE('',#1150,#1036,#793,.T.);
#1409=EDGE_CURVE('',#1152,#1152,#652,.T.);
#1410=EDGE_CURVE('',#1153,#1153,#653,.T.);
#1411=EDGE_CURVE('',#1152,#1023,#794,.T.);
#1412=EDGE_CURVE('',#1154,#1154,#654,.T.);
#1413=EDGE_CURVE('',#1155,#1155,#655,.T.);
#1414=EDGE_CURVE('',#1154,#1041,#795,.T.);
#1415=EDGE_CURVE('',#1156,#1156,#656,.T.);
#1416=EDGE_CURVE('',#1157,#1157,#657,.T.);
#1417=EDGE_CURVE('',#1156,#1026,#796,.T.);
#1418=EDGE_CURVE('',#1158,#1158,#658,.T.);
#1419=EDGE_CURVE('',#1159,#1159,#659,.T.);
#1420=EDGE_CURVE('',#1158,#1044,#797,.T.);
#1421=EDGE_CURVE('',#1129,#1160,#798,.T.);
#1422=EDGE_CURVE('',#1160,#1160,#660,.F.);
#1423=EDGE_CURVE('',#1127,#1161,#799,.T.);
#1424=EDGE_CURVE('',#1161,#1161,#661,.F.);
#1425=EDGE_CURVE('',#1125,#1162,#800,.T.);
#1426=EDGE_CURVE('',#1162,#1162,#662,.F.);
#1427=EDGE_CURVE('',#1123,#1163,#801,.T.);
#1428=EDGE_CURVE('',#1163,#1163,#663,.F.);
#1429=EDGE_CURVE('',#1121,#1164,#802,.T.);
#1430=EDGE_CURVE('',#1164,#1164,#664,.F.);
#1431=EDGE_CURVE('',#1119,#1165,#803,.T.);
#1432=EDGE_CURVE('',#1165,#1165,#665,.F.);
#1433=EDGE_CURVE('',#1117,#1166,#804,.T.);
#1434=EDGE_CURVE('',#1166,#1166,#666,.F.);
#1435=EDGE_CURVE('',#1115,#1167,#805,.T.);
#1436=EDGE_CURVE('',#1167,#1167,#667,.F.);
#1437=EDGE_CURVE('',#1168,#1168,#668,.T.);
#1438=EDGE_CURVE('',#1168,#1141,#806,.T.);
#1439=EDGE_CURVE('',#1169,#1169,#669,.T.);
#1440=EDGE_CURVE('',#1169,#1145,#807,.T.);
#1441=EDGE_CURVE('',#1170,#1170,#670,.T.);
#1442=EDGE_CURVE('',#1170,#1149,#808,.T.);
#1443=EDGE_CURVE('',#1171,#1171,#671,.T.);
#1444=EDGE_CURVE('',#1171,#1151,#809,.T.);
#1445=EDGE_CURVE('',#1172,#1172,#672,.T.);
#1446=EDGE_CURVE('',#1172,#1153,#810,.T.);
#1447=EDGE_CURVE('',#1173,#1173,#673,.T.);
#1448=EDGE_CURVE('',#1173,#1155,#811,.T.);
#1449=EDGE_CURVE('',#1174,#1174,#674,.T.);
#1450=EDGE_CURVE('',#1174,#1157,#812,.T.);
#1451=EDGE_CURVE('',#1175,#1175,#675,.T.);
#1452=EDGE_CURVE('',#1175,#1159,#813,.T.);
#1453=EDGE_CURVE('',#1093,#1076,#814,.T.);
#1454=EDGE_CURVE('',#1075,#1094,#815,.F.);
#1455=EDGE_CURVE('',#1176,#1060,#816,.T.);
#1456=EDGE_CURVE('',#1176,#1099,#817,.T.);
#1457=EDGE_CURVE('',#1100,#1177,#818,.F.);
#1458=EDGE_CURVE('',#1177,#1061,#819,.T.);
#1459=EDGE_CURVE('',#1177,#1176,#269,.T.);
#1460=EDGE_CURVE('',#1095,#1074,#820,.T.);
#1461=EDGE_CURVE('',#1073,#1096,#821,.F.);
#1462=EDGE_CURVE('',#1178,#1046,#822,.T.);
#1463=EDGE_CURVE('',#1178,#1146,#823,.T.);
#1464=EDGE_CURVE('',#1147,#1179,#824,.F.);
#1465=EDGE_CURVE('',#1179,#1047,#825,.T.);
#1466=EDGE_CURVE('',#1179,#1178,#270,.T.);
#1467=EDGE_CURVE('',#1091,#1072,#826,.T.);
#1468=EDGE_CURVE('',#1071,#1092,#827,.F.);
#1469=EDGE_CURVE('',#1180,#1028,#828,.T.);
#1470=EDGE_CURVE('',#1180,#1142,#829,.T.);
#1471=EDGE_CURVE('',#1143,#1181,#830,.F.);
#1472=EDGE_CURVE('',#1181,#1029,#831,.T.);
#1473=EDGE_CURVE('',#1181,#1180,#271,.T.);
#1474=EDGE_CURVE('',#1087,#1082,#832,.T.);
#1475=EDGE_CURVE('',#1086,#1083,#833,.T.);
#1476=EDGE_CURVE('',#1089,#1080,#834,.T.);
#1477=EDGE_CURVE('',#1088,#1081,#835,.T.);
#1478=EDGE_CURVE('',#1085,#1078,#836,.T.);
#1479=EDGE_CURVE('',#1084,#1079,#837,.T.);
#1524=ORIENTED_EDGE('',*,*,#1210,.F.);
#1525=ORIENTED_EDGE('',*,*,#1211,.F.);
#1526=ORIENTED_EDGE('',*,*,#1212,.F.);
#1527=ORIENTED_EDGE('',*,*,#1213,.T.);
#1528=ORIENTED_EDGE('',*,*,#1214,.F.);
#1529=ORIENTED_EDGE('',*,*,#1215,.T.);
#1530=ORIENTED_EDGE('',*,*,#1216,.F.);
#1531=ORIENTED_EDGE('',*,*,#1217,.F.);
#1532=ORIENTED_EDGE('',*,*,#1218,.T.);
#1533=ORIENTED_EDGE('',*,*,#1219,.T.);
#1534=ORIENTED_EDGE('',*,*,#1220,.F.);
#1535=ORIENTED_EDGE('',*,*,#1221,.T.);
#1536=ORIENTED_EDGE('',*,*,#1222,.F.);
#1537=ORIENTED_EDGE('',*,*,#1223,.F.);
#1538=ORIENTED_EDGE('',*,*,#1224,.F.);
#1539=ORIENTED_EDGE('',*,*,#1225,.F.);
#1540=ORIENTED_EDGE('',*,*,#1226,.F.);
#1541=ORIENTED_EDGE('',*,*,#1227,.F.);
#1542=ORIENTED_EDGE('',*,*,#1228,.F.);
#1543=ORIENTED_EDGE('',*,*,#1229,.F.);
#1544=ORIENTED_EDGE('',*,*,#1230,.F.);
#1545=ORIENTED_EDGE('',*,*,#1231,.F.);
#1546=ORIENTED_EDGE('',*,*,#1232,.F.);
#1547=ORIENTED_EDGE('',*,*,#1233,.F.);
#1548=ORIENTED_EDGE('',*,*,#1234,.F.);
#1549=ORIENTED_EDGE('',*,*,#1235,.F.);
#1550=ORIENTED_EDGE('',*,*,#1236,.F.);
#1551=ORIENTED_EDGE('',*,*,#1237,.F.);
#1552=ORIENTED_EDGE('',*,*,#1238,.F.);
#1553=ORIENTED_EDGE('',*,*,#1239,.F.);
#1554=ORIENTED_EDGE('',*,*,#1240,.F.);
#1555=ORIENTED_EDGE('',*,*,#1241,.F.);
#1556=ORIENTED_EDGE('',*,*,#1242,.T.);
#1557=ORIENTED_EDGE('',*,*,#1243,.T.);
#1558=ORIENTED_EDGE('',*,*,#1244,.F.);
#1559=ORIENTED_EDGE('',*,*,#1245,.T.);
#1560=ORIENTED_EDGE('',*,*,#1246,.F.);
#1561=ORIENTED_EDGE('',*,*,#1247,.F.);
#1562=ORIENTED_EDGE('',*,*,#1248,.F.);
#1563=ORIENTED_EDGE('',*,*,#1249,.F.);
#1564=ORIENTED_EDGE('',*,*,#1250,.F.);
#1565=ORIENTED_EDGE('',*,*,#1251,.F.);
#1566=ORIENTED_EDGE('',*,*,#1252,.F.);
#1567=ORIENTED_EDGE('',*,*,#1253,.F.);
#1568=ORIENTED_EDGE('',*,*,#1254,.F.);
#1569=ORIENTED_EDGE('',*,*,#1255,.F.);
#1570=ORIENTED_EDGE('',*,*,#1256,.F.);
#1571=ORIENTED_EDGE('',*,*,#1257,.F.);
#1572=ORIENTED_EDGE('',*,*,#1258,.F.);
#1573=ORIENTED_EDGE('',*,*,#1259,.F.);
#1574=ORIENTED_EDGE('',*,*,#1260,.F.);
#1575=ORIENTED_EDGE('',*,*,#1261,.F.);
#1576=ORIENTED_EDGE('',*,*,#1262,.F.);
#1577=ORIENTED_EDGE('',*,*,#1263,.F.);
#1578=ORIENTED_EDGE('',*,*,#1264,.F.);
#1579=ORIENTED_EDGE('',*,*,#1265,.F.);
#1580=ORIENTED_EDGE('',*,*,#1266,.F.);
#1581=ORIENTED_EDGE('',*,*,#1267,.F.);
#1582=ORIENTED_EDGE('',*,*,#1268,.F.);
#1583=ORIENTED_EDGE('',*,*,#1269,.F.);
#1584=ORIENTED_EDGE('',*,*,#1270,.F.);
#1585=ORIENTED_EDGE('',*,*,#1271,.F.);
#1586=ORIENTED_EDGE('',*,*,#1272,.F.);
#1587=ORIENTED_EDGE('',*,*,#1273,.F.);
#1588=ORIENTED_EDGE('',*,*,#1274,.F.);
#1589=ORIENTED_EDGE('',*,*,#1275,.F.);
#1590=ORIENTED_EDGE('',*,*,#1276,.F.);
#1591=ORIENTED_EDGE('',*,*,#1277,.F.);
#1592=ORIENTED_EDGE('',*,*,#1278,.F.);
#1593=ORIENTED_EDGE('',*,*,#1279,.F.);
#1594=ORIENTED_EDGE('',*,*,#1280,.F.);
#1595=ORIENTED_EDGE('',*,*,#1281,.F.);
#1596=ORIENTED_EDGE('',*,*,#1282,.F.);
#1597=ORIENTED_EDGE('',*,*,#1283,.F.);
#1598=ORIENTED_EDGE('',*,*,#1284,.F.);
#1599=ORIENTED_EDGE('',*,*,#1285,.F.);
#1600=ORIENTED_EDGE('',*,*,#1286,.F.);
#1601=ORIENTED_EDGE('',*,*,#1287,.T.);
#1602=ORIENTED_EDGE('',*,*,#1288,.T.);
#1603=ORIENTED_EDGE('',*,*,#1289,.T.);
#1604=ORIENTED_EDGE('',*,*,#1290,.F.);
#1605=ORIENTED_EDGE('',*,*,#1291,.T.);
#1606=ORIENTED_EDGE('',*,*,#1292,.F.);
#1607=ORIENTED_EDGE('',*,*,#1293,.F.);
#1608=ORIENTED_EDGE('',*,*,#1294,.T.);
#1609=ORIENTED_EDGE('',*,*,#1288,.F.);
#1610=ORIENTED_EDGE('',*,*,#1295,.F.);
#1611=ORIENTED_EDGE('',*,*,#1296,.F.);
#1612=ORIENTED_EDGE('',*,*,#1297,.T.);
#1613=ORIENTED_EDGE('',*,*,#1218,.F.);
#1614=ORIENTED_EDGE('',*,*,#1298,.F.);
#1615=ORIENTED_EDGE('',*,*,#1299,.F.);
#1616=ORIENTED_EDGE('',*,*,#1300,.T.);
#1617=ORIENTED_EDGE('',*,*,#1242,.F.);
#1618=ORIENTED_EDGE('',*,*,#1301,.F.);
#1619=ORIENTED_EDGE('',*,*,#1302,.F.);
#1620=ORIENTED_EDGE('',*,*,#1303,.T.);
#1621=ORIENTED_EDGE('',*,*,#1304,.F.);
#1622=ORIENTED_EDGE('',*,*,#1211,.T.);
#1623=ORIENTED_EDGE('',*,*,#1305,.F.);
#1624=ORIENTED_EDGE('',*,*,#1306,.F.);
#1625=ORIENTED_EDGE('',*,*,#1307,.F.);
#1626=ORIENTED_EDGE('',*,*,#1217,.T.);
#1627=ORIENTED_EDGE('',*,*,#1308,.F.);
#1628=ORIENTED_EDGE('',*,*,#1309,.F.);
#1629=ORIENTED_EDGE('',*,*,#1310,.F.);
#1630=ORIENTED_EDGE('',*,*,#1293,.T.);
#1631=ORIENTED_EDGE('',*,*,#1311,.F.);
#1632=ORIENTED_EDGE('',*,*,#1312,.F.);
#1633=ORIENTED_EDGE('',*,*,#1313,.F.);
#1634=ORIENTED_EDGE('',*,*,#1304,.T.);
#1635=ORIENTED_EDGE('',*,*,#1314,.T.);
#1636=ORIENTED_EDGE('',*,*,#1294,.F.);
#1637=ORIENTED_EDGE('',*,*,#1314,.F.);
#1638=ORIENTED_EDGE('',*,*,#1215,.F.);
#1639=ORIENTED_EDGE('',*,*,#1315,.T.);
#1640=ORIENTED_EDGE('',*,*,#1316,.T.);
#1641=ORIENTED_EDGE('',*,*,#1317,.T.);
#1642=ORIENTED_EDGE('',*,*,#1213,.F.);
#1643=ORIENTED_EDGE('',*,*,#1318,.T.);
#1644=ORIENTED_EDGE('',*,*,#1319,.T.);
#1645=ORIENTED_EDGE('',*,*,#1320,.T.);
#1646=ORIENTED_EDGE('',*,*,#1291,.F.);
#1647=ORIENTED_EDGE('',*,*,#1321,.T.);
#1648=ORIENTED_EDGE('',*,*,#1322,.T.);
#1649=ORIENTED_EDGE('',*,*,#1323,.T.);
#1650=ORIENTED_EDGE('',*,*,#1324,.F.);
#1651=ORIENTED_EDGE('',*,*,#1325,.F.);
#1652=ORIENTED_EDGE('',*,*,#1326,.F.);
#1653=ORIENTED_EDGE('',*,*,#1327,.F.);
#1654=ORIENTED_EDGE('',*,*,#1286,.T.);
#1655=ORIENTED_EDGE('',*,*,#1328,.F.);
#1656=ORIENTED_EDGE('',*,*,#1329,.F.);
#1657=ORIENTED_EDGE('',*,*,#1330,.F.);
#1658=ORIENTED_EDGE('',*,*,#1244,.T.);
#1659=ORIENTED_EDGE('',*,*,#1331,.F.);
#1660=ORIENTED_EDGE('',*,*,#1332,.F.);
#1661=ORIENTED_EDGE('',*,*,#1333,.F.);
#1662=ORIENTED_EDGE('',*,*,#1220,.T.);
#1663=ORIENTED_EDGE('',*,*,#1334,.F.);
#1664=ORIENTED_EDGE('',*,*,#1335,.F.);
#1665=ORIENTED_EDGE('',*,*,#1334,.T.);
#1666=ORIENTED_EDGE('',*,*,#1336,.T.);
#1667=ORIENTED_EDGE('',*,*,#1270,.T.);
#1668=ORIENTED_EDGE('',*,*,#1337,.F.);
#1669=ORIENTED_EDGE('',*,*,#1338,.T.);
#1670=ORIENTED_EDGE('',*,*,#1339,.T.);
#1671=ORIENTED_EDGE('',*,*,#1271,.T.);
#1672=ORIENTED_EDGE('',*,*,#1336,.F.);
#1673=ORIENTED_EDGE('',*,*,#1340,.F.);
#1674=ORIENTED_EDGE('',*,*,#1341,.F.);
#1675=ORIENTED_EDGE('',*,*,#1340,.T.);
#1676=ORIENTED_EDGE('',*,*,#1342,.T.);
#1677=ORIENTED_EDGE('',*,*,#1267,.T.);
#1678=ORIENTED_EDGE('',*,*,#1276,.T.);
#1679=ORIENTED_EDGE('',*,*,#1268,.T.);
#1680=ORIENTED_EDGE('',*,*,#1342,.F.);
#1681=ORIENTED_EDGE('',*,*,#1343,.F.);
#1682=ORIENTED_EDGE('',*,*,#1344,.F.);
#1683=ORIENTED_EDGE('',*,*,#1343,.T.);
#1684=ORIENTED_EDGE('',*,*,#1345,.T.);
#1685=ORIENTED_EDGE('',*,*,#1273,.T.);
#1686=ORIENTED_EDGE('',*,*,#1281,.T.);
#1687=ORIENTED_EDGE('',*,*,#1274,.T.);
#1688=ORIENTED_EDGE('',*,*,#1345,.F.);
#1689=ORIENTED_EDGE('',*,*,#1346,.F.);
#1690=ORIENTED_EDGE('',*,*,#1347,.F.);
#1691=ORIENTED_EDGE('',*,*,#1346,.T.);
#1692=ORIENTED_EDGE('',*,*,#1348,.T.);
#1693=ORIENTED_EDGE('',*,*,#1278,.T.);
#1694=ORIENTED_EDGE('',*,*,#1283,.T.);
#1695=ORIENTED_EDGE('',*,*,#1279,.T.);
#1696=ORIENTED_EDGE('',*,*,#1348,.F.);
#1697=ORIENTED_EDGE('',*,*,#1349,.T.);
#1698=ORIENTED_EDGE('',*,*,#1350,.F.);
#1699=ORIENTED_EDGE('',*,*,#1349,.F.);
#1700=ORIENTED_EDGE('',*,*,#1351,.T.);
#1701=ORIENTED_EDGE('',*,*,#1335,.T.);
#1702=ORIENTED_EDGE('',*,*,#1351,.F.);
#1703=ORIENTED_EDGE('',*,*,#1352,.T.);
#1704=ORIENTED_EDGE('',*,*,#1353,.F.);
#1705=ORIENTED_EDGE('',*,*,#1352,.F.);
#1706=ORIENTED_EDGE('',*,*,#1354,.T.);
#1707=ORIENTED_EDGE('',*,*,#1341,.T.);
#1708=ORIENTED_EDGE('',*,*,#1354,.F.);
#1709=ORIENTED_EDGE('',*,*,#1355,.T.);
#1710=ORIENTED_EDGE('',*,*,#1356,.F.);
#1711=ORIENTED_EDGE('',*,*,#1355,.F.);
#1712=ORIENTED_EDGE('',*,*,#1357,.T.);
#1713=ORIENTED_EDGE('',*,*,#1344,.T.);
#1714=ORIENTED_EDGE('',*,*,#1357,.F.);
#1715=ORIENTED_EDGE('',*,*,#1358,.F.);
#1716=ORIENTED_EDGE('',*,*,#1359,.T.);
#1717=ORIENTED_EDGE('',*,*,#1324,.T.);
#1718=ORIENTED_EDGE('',*,*,#1359,.F.);
#1719=ORIENTED_EDGE('',*,*,#1360,.T.);
#1720=ORIENTED_EDGE('',*,*,#1361,.T.);
#1721=ORIENTED_EDGE('',*,*,#1362,.T.);
#1722=ORIENTED_EDGE('',*,*,#1363,.T.);
#1723=ORIENTED_EDGE('',*,*,#1364,.T.);
#1724=ORIENTED_EDGE('',*,*,#1365,.T.);
#1725=ORIENTED_EDGE('',*,*,#1366,.T.);
#1726=ORIENTED_EDGE('',*,*,#1367,.T.);
#1727=ORIENTED_EDGE('',*,*,#1368,.T.);
#1728=ORIENTED_EDGE('',*,*,#1369,.T.);
#1729=ORIENTED_EDGE('',*,*,#1370,.T.);
#1730=ORIENTED_EDGE('',*,*,#1371,.T.);
#1731=ORIENTED_EDGE('',*,*,#1372,.T.);
#1732=ORIENTED_EDGE('',*,*,#1373,.T.);
#1733=ORIENTED_EDGE('',*,*,#1374,.T.);
#1734=ORIENTED_EDGE('',*,*,#1375,.T.);
#1735=ORIENTED_EDGE('',*,*,#1376,.T.);
#1736=ORIENTED_EDGE('',*,*,#1377,.T.);
#1737=ORIENTED_EDGE('',*,*,#1378,.T.);
#1738=ORIENTED_EDGE('',*,*,#1379,.T.);
#1739=ORIENTED_EDGE('',*,*,#1380,.T.);
#1740=ORIENTED_EDGE('',*,*,#1381,.T.);
#1741=ORIENTED_EDGE('',*,*,#1382,.T.);
#1742=ORIENTED_EDGE('',*,*,#1383,.T.);
#1743=ORIENTED_EDGE('',*,*,#1358,.T.);
#1744=ORIENTED_EDGE('',*,*,#1384,.T.);
#1745=ORIENTED_EDGE('',*,*,#1385,.F.);
#1746=ORIENTED_EDGE('',*,*,#1384,.F.);
#1747=ORIENTED_EDGE('',*,*,#1386,.T.);
#1748=ORIENTED_EDGE('',*,*,#1347,.T.);
#1749=ORIENTED_EDGE('',*,*,#1386,.F.);
#1750=ORIENTED_EDGE('',*,*,#1382,.F.);
#1751=ORIENTED_EDGE('',*,*,#1383,.F.);
#1752=ORIENTED_EDGE('',*,*,#1387,.T.);
#1753=ORIENTED_EDGE('',*,*,#1350,.T.);
#1754=ORIENTED_EDGE('',*,*,#1387,.F.);
#1755=ORIENTED_EDGE('',*,*,#1380,.F.);
#1756=ORIENTED_EDGE('',*,*,#1381,.F.);
#1757=ORIENTED_EDGE('',*,*,#1388,.T.);
#1758=ORIENTED_EDGE('',*,*,#1353,.T.);
#1759=ORIENTED_EDGE('',*,*,#1388,.F.);
#1760=ORIENTED_EDGE('',*,*,#1378,.F.);
#1761=ORIENTED_EDGE('',*,*,#1379,.F.);
#1762=ORIENTED_EDGE('',*,*,#1389,.T.);
#1763=ORIENTED_EDGE('',*,*,#1356,.T.);
#1764=ORIENTED_EDGE('',*,*,#1389,.F.);
#1765=ORIENTED_EDGE('',*,*,#1376,.F.);
#1766=ORIENTED_EDGE('',*,*,#1377,.F.);
#1767=ORIENTED_EDGE('',*,*,#1390,.T.);
#1768=ORIENTED_EDGE('',*,*,#1385,.T.);
#1769=ORIENTED_EDGE('',*,*,#1390,.F.);
#1770=ORIENTED_EDGE('',*,*,#1391,.F.);
#1771=ORIENTED_EDGE('',*,*,#1392,.F.);
#1772=ORIENTED_EDGE('',*,*,#1391,.T.);
#1773=ORIENTED_EDGE('',*,*,#1393,.T.);
#1774=ORIENTED_EDGE('',*,*,#1226,.T.);
#1775=ORIENTED_EDGE('',*,*,#1394,.F.);
#1776=ORIENTED_EDGE('',*,*,#1395,.T.);
#1777=ORIENTED_EDGE('',*,*,#1396,.T.);
#1778=ORIENTED_EDGE('',*,*,#1227,.T.);
#1779=ORIENTED_EDGE('',*,*,#1393,.F.);
#1780=ORIENTED_EDGE('',*,*,#1397,.F.);
#1781=ORIENTED_EDGE('',*,*,#1398,.F.);
#1782=ORIENTED_EDGE('',*,*,#1397,.T.);
#1783=ORIENTED_EDGE('',*,*,#1399,.T.);
#1784=ORIENTED_EDGE('',*,*,#1250,.T.);
#1785=ORIENTED_EDGE('',*,*,#1400,.F.);
#1786=ORIENTED_EDGE('',*,*,#1401,.T.);
#1787=ORIENTED_EDGE('',*,*,#1402,.T.);
#1788=ORIENTED_EDGE('',*,*,#1251,.T.);
#1789=ORIENTED_EDGE('',*,*,#1399,.F.);
#1790=ORIENTED_EDGE('',*,*,#1403,.F.);
#1791=ORIENTED_EDGE('',*,*,#1404,.F.);
#1792=ORIENTED_EDGE('',*,*,#1403,.T.);
#1793=ORIENTED_EDGE('',*,*,#1405,.T.);
#1794=ORIENTED_EDGE('',*,*,#1223,.T.);
#1795=ORIENTED_EDGE('',*,*,#1232,.T.);
#1796=ORIENTED_EDGE('',*,*,#1224,.T.);
#1797=ORIENTED_EDGE('',*,*,#1405,.F.);
#1798=ORIENTED_EDGE('',*,*,#1406,.F.);
#1799=ORIENTED_EDGE('',*,*,#1407,.F.);
#1800=ORIENTED_EDGE('',*,*,#1406,.T.);
#1801=ORIENTED_EDGE('',*,*,#1408,.T.);
#1802=ORIENTED_EDGE('',*,*,#1247,.T.);
#1803=ORIENTED_EDGE('',*,*,#1256,.T.);
#1804=ORIENTED_EDGE('',*,*,#1248,.T.);
#1805=ORIENTED_EDGE('',*,*,#1408,.F.);
#1806=ORIENTED_EDGE('',*,*,#1409,.F.);
#1807=ORIENTED_EDGE('',*,*,#1410,.F.);
#1808=ORIENTED_EDGE('',*,*,#1409,.T.);
#1809=ORIENTED_EDGE('',*,*,#1411,.T.);
#1810=ORIENTED_EDGE('',*,*,#1229,.T.);
#1811=ORIENTED_EDGE('',*,*,#1237,.T.);
#1812=ORIENTED_EDGE('',*,*,#1230,.T.);
#1813=ORIENTED_EDGE('',*,*,#1411,.F.);
#1814=ORIENTED_EDGE('',*,*,#1412,.F.);
#1815=ORIENTED_EDGE('',*,*,#1413,.F.);
#1816=ORIENTED_EDGE('',*,*,#1412,.T.);
#1817=ORIENTED_EDGE('',*,*,#1414,.T.);
#1818=ORIENTED_EDGE('',*,*,#1253,.T.);
#1819=ORIENTED_EDGE('',*,*,#1261,.T.);
#1820=ORIENTED_EDGE('',*,*,#1254,.T.);
#1821=ORIENTED_EDGE('',*,*,#1414,.F.);
#1822=ORIENTED_EDGE('',*,*,#1415,.F.);
#1823=ORIENTED_EDGE('',*,*,#1416,.F.);
#1824=ORIENTED_EDGE('',*,*,#1415,.T.);
#1825=ORIENTED_EDGE('',*,*,#1417,.T.);
#1826=ORIENTED_EDGE('',*,*,#1234,.T.);
#1827=ORIENTED_EDGE('',*,*,#1239,.T.);
#1828=ORIENTED_EDGE('',*,*,#1235,.T.);
#1829=ORIENTED_EDGE('',*,*,#1417,.F.);
#1830=ORIENTED_EDGE('',*,*,#1418,.F.);
#1831=ORIENTED_EDGE('',*,*,#1419,.F.);
#1832=ORIENTED_EDGE('',*,*,#1418,.T.);
#1833=ORIENTED_EDGE('',*,*,#1420,.T.);
#1834=ORIENTED_EDGE('',*,*,#1258,.T.);
#1835=ORIENTED_EDGE('',*,*,#1263,.T.);
#1836=ORIENTED_EDGE('',*,*,#1259,.T.);
#1837=ORIENTED_EDGE('',*,*,#1420,.F.);
#1838=ORIENTED_EDGE('',*,*,#1374,.F.);
#1839=ORIENTED_EDGE('',*,*,#1375,.F.);
#1840=ORIENTED_EDGE('',*,*,#1421,.T.);
#1841=ORIENTED_EDGE('',*,*,#1422,.F.);
#1842=ORIENTED_EDGE('',*,*,#1421,.F.);
#1843=ORIENTED_EDGE('',*,*,#1372,.F.);
#1844=ORIENTED_EDGE('',*,*,#1373,.F.);
#1845=ORIENTED_EDGE('',*,*,#1423,.T.);
#1846=ORIENTED_EDGE('',*,*,#1424,.F.);
#1847=ORIENTED_EDGE('',*,*,#1423,.F.);
#1848=ORIENTED_EDGE('',*,*,#1370,.F.);
#1849=ORIENTED_EDGE('',*,*,#1371,.F.);
#1850=ORIENTED_EDGE('',*,*,#1425,.T.);
#1851=ORIENTED_EDGE('',*,*,#1426,.F.);
#1852=ORIENTED_EDGE('',*,*,#1425,.F.);
#1853=ORIENTED_EDGE('',*,*,#1368,.F.);
#1854=ORIENTED_EDGE('',*,*,#1369,.F.);
#1855=ORIENTED_EDGE('',*,*,#1427,.T.);
#1856=ORIENTED_EDGE('',*,*,#1428,.F.);
#1857=ORIENTED_EDGE('',*,*,#1427,.F.);
#1858=ORIENTED_EDGE('',*,*,#1366,.F.);
#1859=ORIENTED_EDGE('',*,*,#1367,.F.);
#1860=ORIENTED_EDGE('',*,*,#1429,.T.);
#1861=ORIENTED_EDGE('',*,*,#1430,.F.);
#1862=ORIENTED_EDGE('',*,*,#1429,.F.);
#1863=ORIENTED_EDGE('',*,*,#1364,.F.);
#1864=ORIENTED_EDGE('',*,*,#1365,.F.);
#1865=ORIENTED_EDGE('',*,*,#1431,.T.);
#1866=ORIENTED_EDGE('',*,*,#1432,.F.);
#1867=ORIENTED_EDGE('',*,*,#1431,.F.);
#1868=ORIENTED_EDGE('',*,*,#1362,.F.);
#1869=ORIENTED_EDGE('',*,*,#1363,.F.);
#1870=ORIENTED_EDGE('',*,*,#1433,.T.);
#1871=ORIENTED_EDGE('',*,*,#1434,.F.);
#1872=ORIENTED_EDGE('',*,*,#1433,.F.);
#1873=ORIENTED_EDGE('',*,*,#1360,.F.);
#1874=ORIENTED_EDGE('',*,*,#1361,.F.);
#1875=ORIENTED_EDGE('',*,*,#1435,.T.);
#1876=ORIENTED_EDGE('',*,*,#1436,.F.);
#1877=ORIENTED_EDGE('',*,*,#1435,.F.);
#1878=ORIENTED_EDGE('',*,*,#1437,.T.);
#1879=ORIENTED_EDGE('',*,*,#1424,.T.);
#1880=ORIENTED_EDGE('',*,*,#1437,.F.);
#1881=ORIENTED_EDGE('',*,*,#1438,.T.);
#1882=ORIENTED_EDGE('',*,*,#1392,.T.);
#1883=ORIENTED_EDGE('',*,*,#1438,.F.);
#1884=ORIENTED_EDGE('',*,*,#1439,.T.);
#1885=ORIENTED_EDGE('',*,*,#1422,.T.);
#1886=ORIENTED_EDGE('',*,*,#1439,.F.);
#1887=ORIENTED_EDGE('',*,*,#1440,.T.);
#1888=ORIENTED_EDGE('',*,*,#1398,.T.);
#1889=ORIENTED_EDGE('',*,*,#1440,.F.);
#1890=ORIENTED_EDGE('',*,*,#1441,.T.);
#1891=ORIENTED_EDGE('',*,*,#1428,.T.);
#1892=ORIENTED_EDGE('',*,*,#1441,.F.);
#1893=ORIENTED_EDGE('',*,*,#1442,.T.);
#1894=ORIENTED_EDGE('',*,*,#1404,.T.);
#1895=ORIENTED_EDGE('',*,*,#1442,.F.);
#1896=ORIENTED_EDGE('',*,*,#1443,.T.);
#1897=ORIENTED_EDGE('',*,*,#1426,.T.);
#1898=ORIENTED_EDGE('',*,*,#1443,.F.);
#1899=ORIENTED_EDGE('',*,*,#1444,.T.);
#1900=ORIENTED_EDGE('',*,*,#1407,.T.);
#1901=ORIENTED_EDGE('',*,*,#1444,.F.);
#1902=ORIENTED_EDGE('',*,*,#1445,.T.);
#1903=ORIENTED_EDGE('',*,*,#1432,.T.);
#1904=ORIENTED_EDGE('',*,*,#1445,.F.);
#1905=ORIENTED_EDGE('',*,*,#1446,.T.);
#1906=ORIENTED_EDGE('',*,*,#1410,.T.);
#1907=ORIENTED_EDGE('',*,*,#1446,.F.);
#1908=ORIENTED_EDGE('',*,*,#1447,.T.);
#1909=ORIENTED_EDGE('',*,*,#1430,.T.);
#1910=ORIENTED_EDGE('',*,*,#1447,.F.);
#1911=ORIENTED_EDGE('',*,*,#1448,.T.);
#1912=ORIENTED_EDGE('',*,*,#1413,.T.);
#1913=ORIENTED_EDGE('',*,*,#1448,.F.);
#1914=ORIENTED_EDGE('',*,*,#1449,.T.);
#1915=ORIENTED_EDGE('',*,*,#1436,.T.);
#1916=ORIENTED_EDGE('',*,*,#1449,.F.);
#1917=ORIENTED_EDGE('',*,*,#1450,.T.);
#1918=ORIENTED_EDGE('',*,*,#1416,.T.);
#1919=ORIENTED_EDGE('',*,*,#1450,.F.);
#1920=ORIENTED_EDGE('',*,*,#1451,.T.);
#1921=ORIENTED_EDGE('',*,*,#1434,.T.);
#1922=ORIENTED_EDGE('',*,*,#1451,.F.);
#1923=ORIENTED_EDGE('',*,*,#1452,.T.);
#1924=ORIENTED_EDGE('',*,*,#1419,.T.);
#1925=ORIENTED_EDGE('',*,*,#1452,.F.);
#1926=ORIENTED_EDGE('',*,*,#1303,.F.);
#1927=ORIENTED_EDGE('',*,*,#1453,.F.);
#1928=ORIENTED_EDGE('',*,*,#1328,.T.);
#1929=ORIENTED_EDGE('',*,*,#1289,.F.);
#1930=ORIENTED_EDGE('',*,*,#1330,.T.);
#1931=ORIENTED_EDGE('',*,*,#1454,.F.);
#1932=ORIENTED_EDGE('',*,*,#1301,.T.);
#1933=ORIENTED_EDGE('',*,*,#1245,.F.);
#1934=ORIENTED_EDGE('',*,*,#1269,.T.);
#1935=ORIENTED_EDGE('',*,*,#1275,.T.);
#1936=ORIENTED_EDGE('',*,*,#1280,.T.);
#1937=ORIENTED_EDGE('',*,*,#1282,.T.);
#1938=ORIENTED_EDGE('',*,*,#1455,.F.);
#1939=ORIENTED_EDGE('',*,*,#1456,.T.);
#1940=ORIENTED_EDGE('',*,*,#1337,.T.);
#1941=ORIENTED_EDGE('',*,*,#1284,.T.);
#1942=ORIENTED_EDGE('',*,*,#1277,.T.);
#1943=ORIENTED_EDGE('',*,*,#1272,.T.);
#1944=ORIENTED_EDGE('',*,*,#1266,.T.);
#1945=ORIENTED_EDGE('',*,*,#1339,.F.);
#1946=ORIENTED_EDGE('',*,*,#1457,.T.);
#1947=ORIENTED_EDGE('',*,*,#1458,.T.);
#1948=ORIENTED_EDGE('',*,*,#1285,.T.);
#1949=ORIENTED_EDGE('',*,*,#1458,.F.);
#1950=ORIENTED_EDGE('',*,*,#1459,.T.);
#1951=ORIENTED_EDGE('',*,*,#1455,.T.);
#1952=ORIENTED_EDGE('',*,*,#1329,.T.);
#1953=ORIENTED_EDGE('',*,*,#1453,.T.);
#1954=ORIENTED_EDGE('',*,*,#1302,.T.);
#1955=ORIENTED_EDGE('',*,*,#1454,.T.);
#1956=ORIENTED_EDGE('',*,*,#1457,.F.);
#1957=ORIENTED_EDGE('',*,*,#1338,.F.);
#1958=ORIENTED_EDGE('',*,*,#1456,.F.);
#1959=ORIENTED_EDGE('',*,*,#1459,.F.);
#1960=ORIENTED_EDGE('',*,*,#1300,.F.);
#1961=ORIENTED_EDGE('',*,*,#1460,.F.);
#1962=ORIENTED_EDGE('',*,*,#1331,.T.);
#1963=ORIENTED_EDGE('',*,*,#1243,.F.);
#1964=ORIENTED_EDGE('',*,*,#1333,.T.);
#1965=ORIENTED_EDGE('',*,*,#1461,.F.);
#1966=ORIENTED_EDGE('',*,*,#1298,.T.);
#1967=ORIENTED_EDGE('',*,*,#1221,.F.);
#1968=ORIENTED_EDGE('',*,*,#1249,.T.);
#1969=ORIENTED_EDGE('',*,*,#1255,.T.);
#1970=ORIENTED_EDGE('',*,*,#1260,.T.);
#1971=ORIENTED_EDGE('',*,*,#1262,.T.);
#1972=ORIENTED_EDGE('',*,*,#1462,.F.);
#1973=ORIENTED_EDGE('',*,*,#1463,.T.);
#1974=ORIENTED_EDGE('',*,*,#1400,.T.);
#1975=ORIENTED_EDGE('',*,*,#1264,.T.);
#1976=ORIENTED_EDGE('',*,*,#1257,.T.);
#1977=ORIENTED_EDGE('',*,*,#1252,.T.);
#1978=ORIENTED_EDGE('',*,*,#1246,.T.);
#1979=ORIENTED_EDGE('',*,*,#1402,.F.);
#1980=ORIENTED_EDGE('',*,*,#1464,.T.);
#1981=ORIENTED_EDGE('',*,*,#1465,.T.);
#1982=ORIENTED_EDGE('',*,*,#1265,.T.);
#1983=ORIENTED_EDGE('',*,*,#1465,.F.);
#1984=ORIENTED_EDGE('',*,*,#1466,.T.);
#1985=ORIENTED_EDGE('',*,*,#1462,.T.);
#1986=ORIENTED_EDGE('',*,*,#1332,.T.);
#1987=ORIENTED_EDGE('',*,*,#1460,.T.);
#1988=ORIENTED_EDGE('',*,*,#1299,.T.);
#1989=ORIENTED_EDGE('',*,*,#1461,.T.);
#1990=ORIENTED_EDGE('',*,*,#1464,.F.);
#1991=ORIENTED_EDGE('',*,*,#1401,.F.);
#1992=ORIENTED_EDGE('',*,*,#1463,.F.);
#1993=ORIENTED_EDGE('',*,*,#1466,.F.);
#1994=ORIENTED_EDGE('',*,*,#1297,.F.);
#1995=ORIENTED_EDGE('',*,*,#1467,.F.);
#1996=ORIENTED_EDGE('',*,*,#1325,.T.);
#1997=ORIENTED_EDGE('',*,*,#1219,.F.);
#1998=ORIENTED_EDGE('',*,*,#1327,.T.);
#1999=ORIENTED_EDGE('',*,*,#1468,.F.);
#2000=ORIENTED_EDGE('',*,*,#1295,.T.);
#2001=ORIENTED_EDGE('',*,*,#1287,.F.);
#2002=ORIENTED_EDGE('',*,*,#1225,.T.);
#2003=ORIENTED_EDGE('',*,*,#1231,.T.);
#2004=ORIENTED_EDGE('',*,*,#1236,.T.);
#2005=ORIENTED_EDGE('',*,*,#1238,.T.);
#2006=ORIENTED_EDGE('',*,*,#1469,.F.);
#2007=ORIENTED_EDGE('',*,*,#1470,.T.);
#2008=ORIENTED_EDGE('',*,*,#1394,.T.);
#2009=ORIENTED_EDGE('',*,*,#1240,.T.);
#2010=ORIENTED_EDGE('',*,*,#1233,.T.);
#2011=ORIENTED_EDGE('',*,*,#1228,.T.);
#2012=ORIENTED_EDGE('',*,*,#1222,.T.);
#2013=ORIENTED_EDGE('',*,*,#1396,.F.);
#2014=ORIENTED_EDGE('',*,*,#1471,.T.);
#2015=ORIENTED_EDGE('',*,*,#1472,.T.);
#2016=ORIENTED_EDGE('',*,*,#1241,.T.);
#2017=ORIENTED_EDGE('',*,*,#1472,.F.);
#2018=ORIENTED_EDGE('',*,*,#1473,.T.);
#2019=ORIENTED_EDGE('',*,*,#1469,.T.);
#2020=ORIENTED_EDGE('',*,*,#1326,.T.);
#2021=ORIENTED_EDGE('',*,*,#1467,.T.);
#2022=ORIENTED_EDGE('',*,*,#1296,.T.);
#2023=ORIENTED_EDGE('',*,*,#1468,.T.);
#2024=ORIENTED_EDGE('',*,*,#1471,.F.);
#2025=ORIENTED_EDGE('',*,*,#1395,.F.);
#2026=ORIENTED_EDGE('',*,*,#1470,.F.);
#2027=ORIENTED_EDGE('',*,*,#1473,.F.);
#2028=ORIENTED_EDGE('',*,*,#1292,.T.);
#2029=ORIENTED_EDGE('',*,*,#1320,.F.);
#2030=ORIENTED_EDGE('',*,*,#1474,.T.);
#2031=ORIENTED_EDGE('',*,*,#1311,.T.);
#2032=ORIENTED_EDGE('',*,*,#1212,.T.);
#2033=ORIENTED_EDGE('',*,*,#1313,.T.);
#2034=ORIENTED_EDGE('',*,*,#1475,.F.);
#2035=ORIENTED_EDGE('',*,*,#1318,.F.);
#2036=ORIENTED_EDGE('',*,*,#1475,.T.);
#2037=ORIENTED_EDGE('',*,*,#1312,.T.);
#2038=ORIENTED_EDGE('',*,*,#1474,.F.);
#2039=ORIENTED_EDGE('',*,*,#1319,.F.);
#2040=ORIENTED_EDGE('',*,*,#1216,.T.);
#2041=ORIENTED_EDGE('',*,*,#1323,.F.);
#2042=ORIENTED_EDGE('',*,*,#1476,.T.);
#2043=ORIENTED_EDGE('',*,*,#1308,.T.);
#2044=ORIENTED_EDGE('',*,*,#1290,.T.);
#2045=ORIENTED_EDGE('',*,*,#1310,.T.);
#2046=ORIENTED_EDGE('',*,*,#1477,.F.);
#2047=ORIENTED_EDGE('',*,*,#1321,.F.);
#2048=ORIENTED_EDGE('',*,*,#1477,.T.);
#2049=ORIENTED_EDGE('',*,*,#1309,.T.);
#2050=ORIENTED_EDGE('',*,*,#1476,.F.);
#2051=ORIENTED_EDGE('',*,*,#1322,.F.);
#2052=ORIENTED_EDGE('',*,*,#1210,.T.);
#2053=ORIENTED_EDGE('',*,*,#1317,.F.);
#2054=ORIENTED_EDGE('',*,*,#1478,.T.);
#2055=ORIENTED_EDGE('',*,*,#1305,.T.);
#2056=ORIENTED_EDGE('',*,*,#1214,.T.);
#2057=ORIENTED_EDGE('',*,*,#1307,.T.);
#2058=ORIENTED_EDGE('',*,*,#1479,.F.);
#2059=ORIENTED_EDGE('',*,*,#1315,.F.);
#2060=ORIENTED_EDGE('',*,*,#1479,.T.);
#2061=ORIENTED_EDGE('',*,*,#1306,.T.);
#2062=ORIENTED_EDGE('',*,*,#1478,.F.);
#2063=ORIENTED_EDGE('',*,*,#1316,.F.);
#2152=CYLINDRICAL_SURFACE('',#2426,15.);
#2153=CYLINDRICAL_SURFACE('',#2429,15.);
#2154=CYLINDRICAL_SURFACE('',#2432,15.);
#2155=CYLINDRICAL_SURFACE('',#2435,15.);
#2156=CYLINDRICAL_SURFACE('',#2436,15.);
#2157=CYLINDRICAL_SURFACE('',#2437,15.);
#2158=CYLINDRICAL_SURFACE('',#2438,15.);
#2159=CYLINDRICAL_SURFACE('',#2439,15.);
#2160=CYLINDRICAL_SURFACE('',#2442,15.);
#2161=CYLINDRICAL_SURFACE('',#2443,15.);
#2162=CYLINDRICAL_SURFACE('',#2444,15.);
#2163=CYLINDRICAL_SURFACE('',#2445,15.);
#2164=CYLINDRICAL_SURFACE('',#2446,15.);
#2165=CYLINDRICAL_SURFACE('',#2447,15.);
#2166=CYLINDRICAL_SURFACE('',#2448,15.);
#2167=CYLINDRICAL_SURFACE('',#2449,15.);
#2168=CYLINDRICAL_SURFACE('',#2450,15.);
#2169=CYLINDRICAL_SURFACE('',#2453,15.);
#2170=CYLINDRICAL_SURFACE('',#2463,17.);
#2171=CYLINDRICAL_SURFACE('',#2473,4.00000000000012);
#2172=CYLINDRICAL_SURFACE('',#2477,4.00000000000001);
#2173=CYLINDRICAL_SURFACE('',#2481,4.00000000000001);
#2174=CYLINDRICAL_SURFACE('',#2485,4.);
#2175=CYLINDRICAL_SURFACE('',#2489,3.50000000000012);
#2176=CYLINDRICAL_SURFACE('',#2493,3.5);
#2177=CYLINDRICAL_SURFACE('',#2497,3.49999999999992);
#2178=CYLINDRICAL_SURFACE('',#2498,12.9999999999984);
#2179=CYLINDRICAL_SURFACE('',#2504,3.49999999999998);
#2180=CYLINDRICAL_SURFACE('',#2505,2.80000000000012);
#2181=CYLINDRICAL_SURFACE('',#2506,2.79999999999998);
#2182=CYLINDRICAL_SURFACE('',#2507,2.79999999999991);
#2183=CYLINDRICAL_SURFACE('',#2508,2.79999999999999);
#2184=CYLINDRICAL_SURFACE('',#2512,4.00000000000012);
#2185=CYLINDRICAL_SURFACE('',#2516,4.00000000000012);
#2186=CYLINDRICAL_SURFACE('',#2520,4.00000000000001);
#2187=CYLINDRICAL_SURFACE('',#2524,4.00000000000001);
#2188=CYLINDRICAL_SURFACE('',#2528,4.00000000000001);
#2189=CYLINDRICAL_SURFACE('',#2532,4.00000000000001);
#2190=CYLINDRICAL_SURFACE('',#2536,4.);
#2191=CYLINDRICAL_SURFACE('',#2540,4.);
#2192=CYLINDRICAL_SURFACE('',#2541,2.80000000000012);
#2193=CYLINDRICAL_SURFACE('',#2543,2.80000000000012);
#2194=CYLINDRICAL_SURFACE('',#2545,2.79999999999998);
#2195=CYLINDRICAL_SURFACE('',#2547,2.79999999999998);
#2196=CYLINDRICAL_SURFACE('',#2549,2.79999999999991);
#2197=CYLINDRICAL_SURFACE('',#2551,2.79999999999991);
#2198=CYLINDRICAL_SURFACE('',#2553,2.79999999999999);
#2199=CYLINDRICAL_SURFACE('',#2555,2.79999999999999);
#2200=CYLINDRICAL_SURFACE('',#2559,3.50000000000012);
#2201=CYLINDRICAL_SURFACE('',#2562,3.50000000000012);
#2202=CYLINDRICAL_SURFACE('',#2565,3.5);
#2203=CYLINDRICAL_SURFACE('',#2568,3.5);
#2204=CYLINDRICAL_SURFACE('',#2571,3.49999999999992);
#2205=CYLINDRICAL_SURFACE('',#2574,3.49999999999992);
#2206=CYLINDRICAL_SURFACE('',#2577,3.49999999999998);
#2207=CYLINDRICAL_SURFACE('',#2580,3.49999999999998);
#2208=CYLINDRICAL_SURFACE('',#2585,14.5);
#2209=CYLINDRICAL_SURFACE('',#2590,14.5);
#2210=CYLINDRICAL_SURFACE('',#2595,14.5);
#2223=ADVANCED_FACE('',(#272),#2152,.F.);
#2224=ADVANCED_FACE('',(#273),#2153,.F.);
#2225=ADVANCED_FACE('',(#274),#2154,.T.);
#2226=ADVANCED_FACE('',(#275),#2155,.T.);
#2227=ADVANCED_FACE('',(#276),#2156,.T.);
#2228=ADVANCED_FACE('',(#277),#2157,.T.);
#2229=ADVANCED_FACE('',(#278),#2158,.T.);
#2230=ADVANCED_FACE('',(#279),#2159,.T.);
#2231=ADVANCED_FACE('',(#280),#2160,.T.);
#2232=ADVANCED_FACE('',(#281),#2161,.T.);
#2233=ADVANCED_FACE('',(#282),#2162,.T.);
#2234=ADVANCED_FACE('',(#283),#2163,.T.);
#2235=ADVANCED_FACE('',(#284),#2164,.T.);
#2236=ADVANCED_FACE('',(#285),#2165,.T.);
#2237=ADVANCED_FACE('',(#286),#2166,.T.);
#2238=ADVANCED_FACE('',(#287),#2167,.T.);
#2239=ADVANCED_FACE('',(#288),#2168,.T.);
#2240=ADVANCED_FACE('',(#289),#2169,.F.);
#2241=ADVANCED_FACE('',(#290,#90),#144,.T.);
#2242=ADVANCED_FACE('',(#291,#91),#145,.F.);
#2243=ADVANCED_FACE('',(#292),#2170,.T.);
#2244=ADVANCED_FACE('',(#293,#92),#146,.F.);
#2245=ADVANCED_FACE('',(#294),#147,.T.);
#2246=ADVANCED_FACE('',(#295,#93),#148,.F.);
#2247=ADVANCED_FACE('',(#296),#2171,.T.);
#2248=ADVANCED_FACE('',(#297,#94),#149,.F.);
#2249=ADVANCED_FACE('',(#298),#2172,.T.);
#2250=ADVANCED_FACE('',(#299,#95),#150,.F.);
#2251=ADVANCED_FACE('',(#300),#2173,.T.);
#2252=ADVANCED_FACE('',(#301,#96),#151,.F.);
#2253=ADVANCED_FACE('',(#302),#2174,.T.);
#2254=ADVANCED_FACE('',(#303,#97),#152,.T.);
#2255=ADVANCED_FACE('',(#304),#2175,.F.);
#2256=ADVANCED_FACE('',(#305,#98),#153,.T.);
#2257=ADVANCED_FACE('',(#306),#2176,.F.);
#2258=ADVANCED_FACE('',(#307,#99),#154,.T.);
#2259=ADVANCED_FACE('',(#308),#2177,.F.);
#2260=ADVANCED_FACE('',(#309,#100,#101,#102,#103,#104,#105,#106,#107,#108,
#109,#110,#111),#2178,.F.);
#2261=ADVANCED_FACE('',(#310),#155,.F.);
#2262=ADVANCED_FACE('',(#311,#112),#156,.T.);
#2263=ADVANCED_FACE('',(#312),#2179,.F.);
#2264=ADVANCED_FACE('',(#313),#2180,.F.);
#2265=ADVANCED_FACE('',(#314),#2181,.F.);
#2266=ADVANCED_FACE('',(#315),#2182,.F.);
#2267=ADVANCED_FACE('',(#316),#2183,.F.);
#2268=ADVANCED_FACE('',(#317,#113),#157,.F.);
#2269=ADVANCED_FACE('',(#318),#2184,.T.);
#2270=ADVANCED_FACE('',(#319,#114),#158,.F.);
#2271=ADVANCED_FACE('',(#320),#2185,.T.);
#2272=ADVANCED_FACE('',(#321,#115),#159,.F.);
#2273=ADVANCED_FACE('',(#322),#2186,.T.);
#2274=ADVANCED_FACE('',(#323,#116),#160,.F.);
#2275=ADVANCED_FACE('',(#324),#2187,.T.);
#2276=ADVANCED_FACE('',(#325,#117),#161,.F.);
#2277=ADVANCED_FACE('',(#326),#2188,.T.);
#2278=ADVANCED_FACE('',(#327,#118),#162,.F.);
#2279=ADVANCED_FACE('',(#328),#2189,.T.);
#2280=ADVANCED_FACE('',(#329,#119),#163,.F.);
#2281=ADVANCED_FACE('',(#330),#2190,.T.);
#2282=ADVANCED_FACE('',(#331,#120),#164,.F.);
#2283=ADVANCED_FACE('',(#332),#2191,.T.);
#2284=ADVANCED_FACE('',(#333),#2192,.F.);
#2285=ADVANCED_FACE('',(#334),#2193,.F.);
#2286=ADVANCED_FACE('',(#335),#2194,.F.);
#2287=ADVANCED_FACE('',(#336),#2195,.F.);
#2288=ADVANCED_FACE('',(#337),#2196,.F.);
#2289=ADVANCED_FACE('',(#338),#2197,.F.);
#2290=ADVANCED_FACE('',(#339),#2198,.F.);
#2291=ADVANCED_FACE('',(#340),#2199,.F.);
#2292=ADVANCED_FACE('',(#341,#121),#165,.T.);
#2293=ADVANCED_FACE('',(#342),#2200,.F.);
#2294=ADVANCED_FACE('',(#343,#122),#166,.T.);
#2295=ADVANCED_FACE('',(#344),#2201,.F.);
#2296=ADVANCED_FACE('',(#345,#123),#167,.T.);
#2297=ADVANCED_FACE('',(#346),#2202,.F.);
#2298=ADVANCED_FACE('',(#347,#124),#168,.T.);
#2299=ADVANCED_FACE('',(#348),#2203,.F.);
#2300=ADVANCED_FACE('',(#349,#125),#169,.T.);
#2301=ADVANCED_FACE('',(#350),#2204,.F.);
#2302=ADVANCED_FACE('',(#351,#126),#170,.T.);
#2303=ADVANCED_FACE('',(#352),#2205,.F.);
#2304=ADVANCED_FACE('',(#353,#127),#171,.T.);
#2305=ADVANCED_FACE('',(#354),#2206,.F.);
#2306=ADVANCED_FACE('',(#355,#128),#172,.T.);
#2307=ADVANCED_FACE('',(#356),#2207,.F.);
#2308=ADVANCED_FACE('',(#357),#173,.F.);
#2309=ADVANCED_FACE('',(#358),#174,.F.);
#2310=ADVANCED_FACE('',(#359),#175,.T.);
#2311=ADVANCED_FACE('',(#360),#176,.T.);
#2312=ADVANCED_FACE('',(#361),#87,.T.);
#2313=ADVANCED_FACE('',(#362,#129),#2208,.T.);
#2314=ADVANCED_FACE('',(#363),#177,.F.);
#2315=ADVANCED_FACE('',(#364),#178,.F.);
#2316=ADVANCED_FACE('',(#365),#179,.T.);
#2317=ADVANCED_FACE('',(#366),#180,.T.);
#2318=ADVANCED_FACE('',(#367),#88,.T.);
#2319=ADVANCED_FACE('',(#368,#130),#2209,.T.);
#2320=ADVANCED_FACE('',(#369),#181,.F.);
#2321=ADVANCED_FACE('',(#370),#182,.F.);
#2322=ADVANCED_FACE('',(#371),#183,.T.);
#2323=ADVANCED_FACE('',(#372),#184,.T.);
#2324=ADVANCED_FACE('',(#373),#89,.T.);
#2325=ADVANCED_FACE('',(#374,#131),#2210,.T.);
#2326=ADVANCED_FACE('',(#375),#185,.F.);
#2327=ADVANCED_FACE('',(#376),#186,.F.);
#2328=ADVANCED_FACE('',(#377),#187,.F.);
#2329=ADVANCED_FACE('',(#378),#188,.F.);
#2330=ADVANCED_FACE('',(#379),#189,.F.);
#2331=ADVANCED_FACE('',(#380),#190,.F.);
#2332=ADVANCED_FACE('',(#381),#191,.F.);
#2333=ADVANCED_FACE('',(#382),#192,.F.);
#2334=ADVANCED_FACE('',(#383),#193,.F.);
#2363=CLOSED_SHELL('',(#2223,#2224,#2225,#2226,#2227,#2228,#2229,#2230,
#2231,#2232,#2233,#2234,#2235,#2236,#2237,#2238,#2239,#2240,#2241,#2242,
#2243,#2244,#2245,#2246,#2247,#2248,#2249,#2250,#2251,#2252,#2253,#2254,
#2255,#2256,#2257,#2258,#2259,#2260,#2261,#2262,#2263,#2264,#2265,#2266,
#2267,#2268,#2269,#2270,#2271,#2272,#2273,#2274,#2275,#2276,#2277,#2278,
#2279,#2280,#2281,#2282,#2283,#2284,#2285,#2286,#2287,#2288,#2289,#2290,
#2291,#2292,#2293,#2294,#2295,#2296,#2297,#2298,#2299,#2300,#2301,#2302,
#2303,#2304,#2305,#2306,#2307,#2308,#2309,#2310,#2311,#2312,#2313,#2314,
#2315,#2316,#2317,#2318,#2319,#2320,#2321,#2322,#2323,#2324,#2325,#2326,
#2327,#2328,#2329,#2330,#2331,#2332,#2333,#2334));
#2425=AXIS2_PLACEMENT_3D('',#3337,#2680,#2681);
#2426=AXIS2_PLACEMENT_3D('',#3338,#2682,#2683);
#2427=AXIS2_PLACEMENT_3D('',#3343,#2685,#2686);
#2428=AXIS2_PLACEMENT_3D('',#3346,#2688,#2689);
#2429=AXIS2_PLACEMENT_3D('',#3347,#2690,#2691);
#2430=AXIS2_PLACEMENT_3D('',#3352,#2693,#2694);
#2431=AXIS2_PLACEMENT_3D('',#3355,#2696,#2697);
#2432=AXIS2_PLACEMENT_3D('',#3356,#2698,#2699);
#2433=AXIS2_PLACEMENT_3D('',#3359,#2700,#2701);
#2434=AXIS2_PLACEMENT_3D('',#3363,#2703,#2704);
#2435=AXIS2_PLACEMENT_3D('',#3365,#2706,#2707);
#2436=AXIS2_PLACEMENT_3D('',#3418,#2710,#2711);
#2437=AXIS2_PLACEMENT_3D('',#3464,#2714,#2715);
#2438=AXIS2_PLACEMENT_3D('',#3510,#2718,#2719);
#2439=AXIS2_PLACEMENT_3D('',#3563,#2722,#2723);
#2440=AXIS2_PLACEMENT_3D('',#3566,#2724,#2725);
#2441=AXIS2_PLACEMENT_3D('',#3570,#2727,#2728);
#2442=AXIS2_PLACEMENT_3D('',#3572,#2730,#2731);
#2443=AXIS2_PLACEMENT_3D('',#3625,#2734,#2735);
#2444=AXIS2_PLACEMENT_3D('',#3671,#2738,#2739);
#2445=AXIS2_PLACEMENT_3D('',#3717,#2742,#2743);
#2446=AXIS2_PLACEMENT_3D('',#3770,#2746,#2747);
#2447=AXIS2_PLACEMENT_3D('',#3823,#2750,#2751);
#2448=AXIS2_PLACEMENT_3D('',#3869,#2754,#2755);
#2449=AXIS2_PLACEMENT_3D('',#3915,#2758,#2759);
#2450=AXIS2_PLACEMENT_3D('',#3968,#2762,#2763);
#2451=AXIS2_PLACEMENT_3D('',#3971,#2764,#2765);
#2452=AXIS2_PLACEMENT_3D('',#3975,#2767,#2768);
#2453=AXIS2_PLACEMENT_3D('',#3977,#2770,#2771);
#2454=AXIS2_PLACEMENT_3D('',#3982,#2773,#2774);
#2455=AXIS2_PLACEMENT_3D('',#3985,#2776,#2777);
#2456=AXIS2_PLACEMENT_3D('',#3986,#2778,#2779);
#2457=AXIS2_PLACEMENT_3D('',#3988,#2780,#2781);
#2458=AXIS2_PLACEMENT_3D('',#3992,#2783,#2784);
#2459=AXIS2_PLACEMENT_3D('',#3997,#2787,#2788);
#2460=AXIS2_PLACEMENT_3D('',#4002,#2791,#2792);
#2461=AXIS2_PLACEMENT_3D('',#4004,#2794,#2795);
#2462=AXIS2_PLACEMENT_3D('',#4006,#2796,#2797);
#2463=AXIS2_PLACEMENT_3D('',#4022,#2807,#2808);
#2464=AXIS2_PLACEMENT_3D('',#4024,#2810,#2811);
#2465=AXIS2_PLACEMENT_3D('',#4041,#2821,#2822);
#2466=AXIS2_PLACEMENT_3D('',#4042,#2823,#2824);
#2467=AXIS2_PLACEMENT_3D('',#4046,#2826,#2827);
#2468=AXIS2_PLACEMENT_3D('',#4051,#2830,#2831);
#2469=AXIS2_PLACEMENT_3D('',#4056,#2834,#2835);
#2470=AXIS2_PLACEMENT_3D('',#4058,#2837,#2838);
#2471=AXIS2_PLACEMENT_3D('',#4060,#2839,#2840);
#2472=AXIS2_PLACEMENT_3D('',#4062,#2841,#2842);
#2473=AXIS2_PLACEMENT_3D('',#4063,#2843,#2844);
#2474=AXIS2_PLACEMENT_3D('',#4087,#2848,#2849);
#2475=AXIS2_PLACEMENT_3D('',#4089,#2850,#2851);
#2476=AXIS2_PLACEMENT_3D('',#4091,#2852,#2853);
#2477=AXIS2_PLACEMENT_3D('',#4092,#2854,#2855);
#2478=AXIS2_PLACEMENT_3D('',#4094,#2857,#2858);
#2479=AXIS2_PLACEMENT_3D('',#4096,#2859,#2860);
#2480=AXIS2_PLACEMENT_3D('',#4098,#2861,#2862);
#2481=AXIS2_PLACEMENT_3D('',#4099,#2863,#2864);
#2482=AXIS2_PLACEMENT_3D('',#4101,#2866,#2867);
#2483=AXIS2_PLACEMENT_3D('',#4103,#2868,#2869);
#2484=AXIS2_PLACEMENT_3D('',#4105,#2870,#2871);
#2485=AXIS2_PLACEMENT_3D('',#4106,#2872,#2873);
#2486=AXIS2_PLACEMENT_3D('',#4108,#2875,#2876);
#2487=AXIS2_PLACEMENT_3D('',#4110,#2877,#2878);
#2488=AXIS2_PLACEMENT_3D('',#4112,#2879,#2880);
#2489=AXIS2_PLACEMENT_3D('',#4113,#2881,#2882);
#2490=AXIS2_PLACEMENT_3D('',#4115,#2884,#2885);
#2491=AXIS2_PLACEMENT_3D('',#4117,#2886,#2887);
#2492=AXIS2_PLACEMENT_3D('',#4119,#2888,#2889);
#2493=AXIS2_PLACEMENT_3D('',#4120,#2890,#2891);
#2494=AXIS2_PLACEMENT_3D('',#4122,#2893,#2894);
#2495=AXIS2_PLACEMENT_3D('',#4124,#2895,#2896);
#2496=AXIS2_PLACEMENT_3D('',#4126,#2897,#2898);
#2497=AXIS2_PLACEMENT_3D('',#4127,#2899,#2900);
#2498=AXIS2_PLACEMENT_3D('',#4129,#2902,#2903);
#2499=AXIS2_PLACEMENT_3D('',#4131,#2904,#2905);
#2500=AXIS2_PLACEMENT_3D('',#4661,#2907,#2908);
#2501=AXIS2_PLACEMENT_3D('',#4662,#2909,#2910);
#2502=AXIS2_PLACEMENT_3D('',#4664,#2911,#2912);
#2503=AXIS2_PLACEMENT_3D('',#4666,#2913,#2914);
#2504=AXIS2_PLACEMENT_3D('',#4667,#2915,#2916);
#2505=AXIS2_PLACEMENT_3D('',#4669,#2918,#2919);
#2506=AXIS2_PLACEMENT_3D('',#4671,#2921,#2922);
#2507=AXIS2_PLACEMENT_3D('',#4673,#2924,#2925);
#2508=AXIS2_PLACEMENT_3D('',#4675,#2927,#2928);
#2509=AXIS2_PLACEMENT_3D('',#4677,#2930,#2931);
#2510=AXIS2_PLACEMENT_3D('',#4679,#2932,#2933);
#2511=AXIS2_PLACEMENT_3D('',#4681,#2934,#2935);
#2512=AXIS2_PLACEMENT_3D('',#4682,#2936,#2937);
#2513=AXIS2_PLACEMENT_3D('',#4706,#2941,#2942);
#2514=AXIS2_PLACEMENT_3D('',#4708,#2943,#2944);
#2515=AXIS2_PLACEMENT_3D('',#4710,#2945,#2946);
#2516=AXIS2_PLACEMENT_3D('',#4711,#2947,#2948);
#2517=AXIS2_PLACEMENT_3D('',#4735,#2952,#2953);
#2518=AXIS2_PLACEMENT_3D('',#4737,#2954,#2955);
#2519=AXIS2_PLACEMENT_3D('',#4739,#2956,#2957);
#2520=AXIS2_PLACEMENT_3D('',#4740,#2958,#2959);
#2521=AXIS2_PLACEMENT_3D('',#4742,#2961,#2962);
#2522=AXIS2_PLACEMENT_3D('',#4744,#2963,#2964);
#2523=AXIS2_PLACEMENT_3D('',#4746,#2965,#2966);
#2524=AXIS2_PLACEMENT_3D('',#4747,#2967,#2968);
#2525=AXIS2_PLACEMENT_3D('',#4749,#2970,#2971);
#2526=AXIS2_PLACEMENT_3D('',#4751,#2972,#2973);
#2527=AXIS2_PLACEMENT_3D('',#4753,#2974,#2975);
#2528=AXIS2_PLACEMENT_3D('',#4754,#2976,#2977);
#2529=AXIS2_PLACEMENT_3D('',#4756,#2979,#2980);
#2530=AXIS2_PLACEMENT_3D('',#4758,#2981,#2982);
#2531=AXIS2_PLACEMENT_3D('',#4760,#2983,#2984);
#2532=AXIS2_PLACEMENT_3D('',#4761,#2985,#2986);
#2533=AXIS2_PLACEMENT_3D('',#4763,#2988,#2989);
#2534=AXIS2_PLACEMENT_3D('',#4765,#2990,#2991);
#2535=AXIS2_PLACEMENT_3D('',#4767,#2992,#2993);
#2536=AXIS2_PLACEMENT_3D('',#4768,#2994,#2995);
#2537=AXIS2_PLACEMENT_3D('',#4770,#2997,#2998);
#2538=AXIS2_PLACEMENT_3D('',#4772,#2999,#3000);
#2539=AXIS2_PLACEMENT_3D('',#4774,#3001,#3002);
#2540=AXIS2_PLACEMENT_3D('',#4775,#3003,#3004);
#2541=AXIS2_PLACEMENT_3D('',#4777,#3006,#3007);
#2542=AXIS2_PLACEMENT_3D('',#4780,#3009,#3010);
#2543=AXIS2_PLACEMENT_3D('',#4781,#3011,#3012);
#2544=AXIS2_PLACEMENT_3D('',#4784,#3014,#3015);
#2545=AXIS2_PLACEMENT_3D('',#4785,#3016,#3017);
#2546=AXIS2_PLACEMENT_3D('',#4788,#3019,#3020);
#2547=AXIS2_PLACEMENT_3D('',#4789,#3021,#3022);
#2548=AXIS2_PLACEMENT_3D('',#4792,#3024,#3025);
#2549=AXIS2_PLACEMENT_3D('',#4793,#3026,#3027);
#2550=AXIS2_PLACEMENT_3D('',#4796,#3029,#3030);
#2551=AXIS2_PLACEMENT_3D('',#4797,#3031,#3032);
#2552=AXIS2_PLACEMENT_3D('',#4800,#3034,#3035);
#2553=AXIS2_PLACEMENT_3D('',#4801,#3036,#3037);
#2554=AXIS2_PLACEMENT_3D('',#4804,#3039,#3040);
#2555=AXIS2_PLACEMENT_3D('',#4805,#3041,#3042);
#2556=AXIS2_PLACEMENT_3D('',#4808,#3044,#3045);
#2557=AXIS2_PLACEMENT_3D('',#4809,#3046,#3047);
#2558=AXIS2_PLACEMENT_3D('',#4811,#3048,#3049);
#2559=AXIS2_PLACEMENT_3D('',#4812,#3050,#3051);
#2560=AXIS2_PLACEMENT_3D('',#4814,#3053,#3054);
#2561=AXIS2_PLACEMENT_3D('',#4816,#3055,#3056);
#2562=AXIS2_PLACEMENT_3D('',#4817,#3057,#3058);
#2563=AXIS2_PLACEMENT_3D('',#4819,#3060,#3061);
#2564=AXIS2_PLACEMENT_3D('',#4821,#3062,#3063);
#2565=AXIS2_PLACEMENT_3D('',#4822,#3064,#3065);
#2566=AXIS2_PLACEMENT_3D('',#4824,#3067,#3068);
#2567=AXIS2_PLACEMENT_3D('',#4826,#3069,#3070);
#2568=AXIS2_PLACEMENT_3D('',#4827,#3071,#3072);
#2569=AXIS2_PLACEMENT_3D('',#4829,#3074,#3075);
#2570=AXIS2_PLACEMENT_3D('',#4831,#3076,#3077);
#2571=AXIS2_PLACEMENT_3D('',#4832,#3078,#3079);
#2572=AXIS2_PLACEMENT_3D('',#4834,#3081,#3082);
#2573=AXIS2_PLACEMENT_3D('',#4836,#3083,#3084);
#2574=AXIS2_PLACEMENT_3D('',#4837,#3085,#3086);
#2575=AXIS2_PLACEMENT_3D('',#4839,#3088,#3089);
#2576=AXIS2_PLACEMENT_3D('',#4841,#3090,#3091);
#2577=AXIS2_PLACEMENT_3D('',#4842,#3092,#3093);
#2578=AXIS2_PLACEMENT_3D('',#4844,#3095,#3096);
#2579=AXIS2_PLACEMENT_3D('',#4846,#3097,#3098);
#2580=AXIS2_PLACEMENT_3D('',#4847,#3099,#3100);
#2581=AXIS2_PLACEMENT_3D('',#4849,#3102,#3103);
#2582=AXIS2_PLACEMENT_3D('',#4851,#3105,#3106);
#2583=AXIS2_PLACEMENT_3D('',#4853,#3108,#3109);
#2584=AXIS2_PLACEMENT_3D('',#4857,#3112,#3113);
#2585=AXIS2_PLACEMENT_3D('',#4911,#3116,#3117);
#2586=AXIS2_PLACEMENT_3D('',#4912,#3118,#3119);
#2587=AXIS2_PLACEMENT_3D('',#4914,#3121,#3122);
#2588=AXIS2_PLACEMENT_3D('',#4916,#3124,#3125);
#2589=AXIS2_PLACEMENT_3D('',#4920,#3128,#3129);
#2590=AXIS2_PLACEMENT_3D('',#4974,#3132,#3133);
#2591=AXIS2_PLACEMENT_3D('',#4975,#3134,#3135);
#2592=AXIS2_PLACEMENT_3D('',#4977,#3137,#3138);
#2593=AXIS2_PLACEMENT_3D('',#4979,#3140,#3141);
#2594=AXIS2_PLACEMENT_3D('',#4983,#3144,#3145);
#2595=AXIS2_PLACEMENT_3D('',#5037,#3148,#3149);
#2596=AXIS2_PLACEMENT_3D('',#5038,#3150,#3151);
#2597=AXIS2_PLACEMENT_3D('',#5040,#3153,#3154);
#2598=AXIS2_PLACEMENT_3D('',#5042,#3156,#3157);
#2599=AXIS2_PLACEMENT_3D('',#5043,#3158,#3159);
#2600=AXIS2_PLACEMENT_3D('',#5045,#3161,#3162);
#2601=AXIS2_PLACEMENT_3D('',#5047,#3164,#3165);
#2602=AXIS2_PLACEMENT_3D('',#5048,#3166,#3167);
#2603=AXIS2_PLACEMENT_3D('',#5050,#3169,#3170);
#2604=AXIS2_PLACEMENT_3D('',#5052,#3172,#3173);
#2680=DIRECTION('axis',(0.,0.,1.));
#2681=DIRECTION('refdir',(1.,0.,0.));
#2682=DIRECTION('center_axis',(0.866025403784443,0.,0.499999999999992));
#2683=DIRECTION('ref_axis',(0.499999999999992,0.,-0.866025403784443));
#2684=DIRECTION('',(0.866025403784444,0.,0.499999999999991));
#2685=DIRECTION('center_axis',(-0.866025403784443,0.,-0.499999999999992));
#2686=DIRECTION('ref_axis',(-0.499999999999992,0.,0.866025403784443));
#2687=DIRECTION('',(0.866025403784443,0.,0.499999999999992));
#2688=DIRECTION('center_axis',(-0.866025403784443,0.,-0.499999999999992));
#2689=DIRECTION('ref_axis',(-0.499999999999992,0.,0.866025403784443));
#2690=DIRECTION('center_axis',(0.866025403784443,0.,0.499999999999992));
#2691=DIRECTION('ref_axis',(0.499999999999992,0.,-0.866025403784443));
#2692=DIRECTION('',(0.866025403784443,0.,0.499999999999993));
#2693=DIRECTION('center_axis',(-0.866025403784443,0.,-0.499999999999992));
#2694=DIRECTION('ref_axis',(-0.499999999999992,0.,0.866025403784443));
#2695=DIRECTION('',(0.866025403784443,0.,0.499999999999993));
#2696=DIRECTION('center_axis',(-0.866025403784443,0.,-0.499999999999992));
#2697=DIRECTION('ref_axis',(-0.499999999999992,0.,0.866025403784443));
#2698=DIRECTION('center_axis',(0.866025403784443,0.,0.499999999999992));
#2699=DIRECTION('ref_axis',(0.499999999999992,0.,-0.866025403784443));
#2700=DIRECTION('center_axis',(-0.866025403784443,0.,-0.499999999999992));
#2701=DIRECTION('ref_axis',(-0.499999999999992,0.,0.866025403784443));
#2702=DIRECTION('',(0.866025403784443,0.,0.499999999999992));
#2703=DIRECTION('center_axis',(-0.866025403784443,0.,-0.499999999999992));
#2704=DIRECTION('ref_axis',(-0.499999999999992,0.,0.866025403784443));
#2705=DIRECTION('',(0.866025403784443,0.,0.499999999999992));
#2706=DIRECTION('center_axis',(0.866025403784443,0.,0.499999999999992));
#2707=DIRECTION('ref_axis',(0.499999999999992,0.,-0.866025403784443));
#2708=DIRECTION('',(0.866025403784443,0.,0.499999999999992));
#2709=DIRECTION('',(0.866025403784443,0.,0.499999999999992));
#2710=DIRECTION('center_axis',(0.866025403784443,0.,0.499999999999992));
#2711=DIRECTION('ref_axis',(0.499999999999992,0.,-0.866025403784443));
#2712=DIRECTION('',(0.866025403784443,0.,0.499999999999992));
#2713=DIRECTION('',(0.866025403784443,0.,0.499999999999992));
#2714=DIRECTION('center_axis',(0.866025403784443,0.,0.499999999999992));
#2715=DIRECTION('ref_axis',(0.499999999999992,0.,-0.866025403784443));
#2716=DIRECTION('',(0.866025403784444,0.,0.499999999999991));
#2717=DIRECTION('',(0.866025403784443,0.,0.499999999999992));
#2718=DIRECTION('center_axis',(0.866025403784443,0.,0.499999999999992));
#2719=DIRECTION('ref_axis',(0.499999999999992,0.,-0.866025403784443));
#2720=DIRECTION('',(0.866025403784443,0.,0.499999999999993));
#2721=DIRECTION('',(0.866025403784443,0.,0.499999999999992));
#2722=DIRECTION('center_axis',(0.866025403784443,0.,0.499999999999992));
#2723=DIRECTION('ref_axis',(0.499999999999992,0.,-0.866025403784443));
#2724=DIRECTION('center_axis',(-0.866025403784443,0.,-0.499999999999992));
#2725=DIRECTION('ref_axis',(-0.499999999999992,0.,0.866025403784443));
#2726=DIRECTION('',(0.866025403784443,0.,0.499999999999992));
#2727=DIRECTION('center_axis',(-0.866025403784443,0.,-0.499999999999992));
#2728=DIRECTION('ref_axis',(-0.499999999999992,0.,0.866025403784443));
#2729=DIRECTION('',(0.866025403784443,0.,0.499999999999992));
#2730=DIRECTION('center_axis',(0.866025403784443,0.,0.499999999999992));
#2731=DIRECTION('ref_axis',(0.499999999999992,0.,-0.866025403784443));
#2732=DIRECTION('',(0.866025403784443,0.,0.499999999999992));
#2733=DIRECTION('',(0.866025403784443,0.,0.499999999999993));
#2734=DIRECTION('center_axis',(0.866025403784443,0.,0.499999999999992));
#2735=DIRECTION('ref_axis',(0.499999999999992,0.,-0.866025403784443));
#2736=DIRECTION('',(0.866025403784444,0.,0.499999999999991));
#2737=DIRECTION('',(0.866025403784443,0.,0.499999999999992));
#2738=DIRECTION('center_axis',(0.866025403784443,0.,0.499999999999992));
#2739=DIRECTION('ref_axis',(0.499999999999992,0.,-0.866025403784443));
#2740=DIRECTION('',(0.866025403784443,0.,0.499999999999992));
#2741=DIRECTION('',(0.866025403784443,0.,0.499999999999992));
#2742=DIRECTION('center_axis',(0.866025403784443,0.,0.499999999999992));
#2743=DIRECTION('ref_axis',(0.499999999999992,0.,-0.866025403784443));
#2744=DIRECTION('',(0.866025403784444,0.,0.49999999999999));
#2745=DIRECTION('',(0.866025403784441,0.,0.499999999999995));
#2746=DIRECTION('center_axis',(0.866025403784443,0.,0.499999999999992));
#2747=DIRECTION('ref_axis',(0.499999999999992,0.,-0.866025403784443));
#2748=DIRECTION('',(0.866025403784443,0.,0.499999999999993));
#2749=DIRECTION('',(0.866025403784443,0.,0.499999999999992));
#2750=DIRECTION('center_axis',(0.866025403784443,0.,0.499999999999992));
#2751=DIRECTION('ref_axis',(0.499999999999992,0.,-0.866025403784443));
#2752=DIRECTION('',(0.866025403784443,0.,0.499999999999992));
#2753=DIRECTION('',(0.866025403784443,0.,0.499999999999992));
#2754=DIRECTION('center_axis',(0.866025403784443,0.,0.499999999999992));
#2755=DIRECTION('ref_axis',(0.499999999999992,0.,-0.866025403784443));
#2756=DIRECTION('',(0.866025403784443,0.,0.499999999999992));
#2757=DIRECTION('',(0.866025403784443,0.,0.499999999999992));
#2758=DIRECTION('center_axis',(0.866025403784443,0.,0.499999999999992));
#2759=DIRECTION('ref_axis',(0.499999999999992,0.,-0.866025403784443));
#2760=DIRECTION('',(0.866025403784443,0.,0.499999999999992));
#2761=DIRECTION('',(0.866025403784444,0.,0.499999999999991));
#2762=DIRECTION('center_axis',(0.866025403784443,0.,0.499999999999992));
#2763=DIRECTION('ref_axis',(-0.433012701892211,0.500000000000004,0.750000000000002));
#2764=DIRECTION('center_axis',(-0.866025403784443,0.,-0.499999999999992));
#2765=DIRECTION('ref_axis',(-0.499999999999992,0.,0.866025403784443));
#2766=DIRECTION('',(0.866025403784443,0.,0.499999999999992));
#2767=DIRECTION('center_axis',(-0.866025403784443,0.,-0.499999999999992));
#2768=DIRECTION('ref_axis',(-0.499999999999992,0.,0.866025403784443));
#2769=DIRECTION('',(0.866025403784443,0.,0.499999999999992));
#2770=DIRECTION('center_axis',(0.866025403784443,0.,0.499999999999992));
#2771=DIRECTION('ref_axis',(-0.433012701892234,0.499999999999926,0.750000000000041));
#2772=DIRECTION('',(0.866025403784443,0.,0.499999999999992));
#2773=DIRECTION('center_axis',(-0.866025403784443,0.,-0.499999999999992));
#2774=DIRECTION('ref_axis',(-0.499999999999992,0.,0.866025403784443));
#2775=DIRECTION('',(0.866025403784442,0.,0.499999999999994));
#2776=DIRECTION('center_axis',(-0.866025403784443,0.,-0.499999999999992));
#2777=DIRECTION('ref_axis',(-0.499999999999992,0.,0.866025403784443));
#2778=DIRECTION('center_axis',(-0.866025403784443,0.,-0.499999999999992));
#2779=DIRECTION('ref_axis',(-0.499999999999992,0.,0.866025403784443));
#2780=DIRECTION('center_axis',(-0.866025403784443,0.,-0.499999999999992));
#2781=DIRECTION('ref_axis',(-0.499999999999992,0.,0.866025403784443));
#2782=DIRECTION('',(-0.433012701892229,-0.499999999999983,0.750000000000006));
#2783=DIRECTION('center_axis',(0.866025403784443,-2.25118642417821E-16,
0.499999999999992));
#2784=DIRECTION('ref_axis',(0.499999999999992,0.,-0.866025403784443));
#2785=DIRECTION('',(-0.433012701892221,-0.499999999999992,0.750000000000004));
#2786=DIRECTION('',(0.433012701892197,-0.500000000000028,-0.749999999999994));
#2787=DIRECTION('center_axis',(0.866025403784443,2.4704687096211E-16,0.499999999999992));
#2788=DIRECTION('ref_axis',(0.499999999999992,0.,-0.866025403784443));
#2789=DIRECTION('',(0.433012701892204,-0.500000000000004,-0.750000000000006));
#2790=DIRECTION('',(0.,1.,0.));
#2791=DIRECTION('center_axis',(0.866025403784443,0.,0.499999999999992));
#2792=DIRECTION('ref_axis',(0.499999999999992,0.,-0.866025403784443));
#2793=DIRECTION('',(0.,1.,0.));
#2794=DIRECTION('center_axis',(-0.866025403784443,0.,-0.499999999999992));
#2795=DIRECTION('ref_axis',(-0.499999999999992,0.,0.866025403784443));
#2796=DIRECTION('center_axis',(-0.866025403784443,0.,-0.499999999999992));
#2797=DIRECTION('ref_axis',(-0.499999999999992,0.,0.866025403784443));
#2798=DIRECTION('',(-0.43301270189221,0.500000000000002,0.750000000000004));
#2799=DIRECTION('',(0.25,0.866025403784439,-0.433012701892219));
#2800=DIRECTION('',(0.433012701892205,-0.500000000000012,-0.75));
#2801=DIRECTION('',(0.433012701892215,0.499999999999987,-0.750000000000011));
#2802=DIRECTION('',(0.25,-0.86602540378444,-0.433012701892216));
#2803=DIRECTION('',(-0.433012701892207,-0.499999999999993,0.750000000000012));
#2804=DIRECTION('',(0.,-1.,0.));
#2805=DIRECTION('',(-0.499999999999994,0.,0.866025403784442));
#2806=DIRECTION('',(0.,1.,0.));
#2807=DIRECTION('center_axis',(0.866025403784443,0.,0.499999999999992));
#2808=DIRECTION('ref_axis',(0.499999999999992,0.,-0.866025403784443));
#2809=DIRECTION('',(-0.866025403784443,0.,-0.499999999999992));
#2810=DIRECTION('center_axis',(-0.866025403784443,0.,-0.499999999999992));
#2811=DIRECTION('ref_axis',(-0.499999999999992,0.,0.866025403784443));
#2812=DIRECTION('',(0.433012701892209,-0.500000000000007,-0.750000000000001));
#2813=DIRECTION('',(0.250000000000001,0.866025403784442,-0.433012701892212));
#2814=DIRECTION('',(-0.433012701892215,0.499999999999997,0.750000000000005));
#2815=DIRECTION('',(0.,1.,0.));
#2816=DIRECTION('',(-0.499999999999994,0.,0.866025403784442));
#2817=DIRECTION('',(0.,-1.,0.));
#2818=DIRECTION('',(-0.433012701892214,-0.499999999999991,0.750000000000009));
#2819=DIRECTION('',(0.249999999999992,-0.866025403784442,-0.433012701892217));
#2820=DIRECTION('',(0.433012701892219,0.499999999999982,-0.750000000000012));
#2821=DIRECTION('center_axis',(0.866025403784443,0.,0.499999999999992));
#2822=DIRECTION('ref_axis',(0.499999999999992,0.,-0.866025403784443));
#2823=DIRECTION('center_axis',(-0.866025403784443,0.,-0.499999999999992));
#2824=DIRECTION('ref_axis',(-0.499999999999992,0.,0.866025403784443));
#2825=DIRECTION('',(-0.433012701892211,-0.49999999999998,0.750000000000018));
#2826=DIRECTION('center_axis',(-0.866025403784443,0.,-0.499999999999992));
#2827=DIRECTION('ref_axis',(-0.499999999999992,0.,0.866025403784443));
#2828=DIRECTION('',(0.433012701892242,0.49999999999998,-0.750000000000001));
#2829=DIRECTION('',(0.,1.,0.));
#2830=DIRECTION('center_axis',(-0.866025403784443,0.,-0.499999999999992));
#2831=DIRECTION('ref_axis',(-0.499999999999992,0.,0.866025403784443));
#2832=DIRECTION('',(0.,-1.,0.));
#2833=DIRECTION('',(0.433012701892204,-0.500000000000004,-0.750000000000006));
#2834=DIRECTION('center_axis',(-0.866025403784443,0.,-0.499999999999992));
#2835=DIRECTION('ref_axis',(-0.499999999999992,0.,0.866025403784443));
#2836=DIRECTION('',(-0.433012701892195,0.499999999999999,0.750000000000015));
#2837=DIRECTION('center_axis',(0.,-1.,0.));
#2838=DIRECTION('ref_axis',(0.,0.,-1.));
#2839=DIRECTION('center_axis',(0.,-1.,0.));
#2840=DIRECTION('ref_axis',(0.,0.,-1.));
#2841=DIRECTION('center_axis',(0.,1.,0.));
#2842=DIRECTION('ref_axis',(0.,0.,1.));
#2843=DIRECTION('center_axis',(0.,1.,0.));
#2844=DIRECTION('ref_axis',(0.,0.,1.));
#2845=DIRECTION('',(0.,-1.,0.));
#2846=DIRECTION('',(0.,1.,0.));
#2847=DIRECTION('',(0.,1.,0.));
#2848=DIRECTION('center_axis',(0.224143868042018,-0.965925826289067,0.129409522551263));
#2849=DIRECTION('ref_axis',(0.,-0.132788176096111,-0.991144439670156));
#2850=DIRECTION('center_axis',(0.224143868042018,-0.965925826289067,0.129409522551263));
#2851=DIRECTION('ref_axis',(0.974116947696296,0.22604462437946,0.));
#2852=DIRECTION('center_axis',(-0.224143868042018,0.965925826289067,-0.129409522551263));
#2853=DIRECTION('ref_axis',(-0.974116947696296,-0.22604462437946,0.));
#2854=DIRECTION('center_axis',(-0.224143868042018,0.965925826289067,-0.129409522551263));
#2855=DIRECTION('ref_axis',(-0.974116947696296,-0.22604462437946,0.));
#2856=DIRECTION('',(0.224143868042018,-0.965925826289067,0.129409522551263));
#2857=DIRECTION('center_axis',(0.433012701892223,-0.866025403784436,0.250000000000002));
#2858=DIRECTION('ref_axis',(0.5,0.,-0.866025403784439));
#2859=DIRECTION('center_axis',(0.433012701892223,-0.866025403784436,0.250000000000002));
#2860=DIRECTION('ref_axis',(0.894427190999914,0.447213595499962,0.));
#2861=DIRECTION('center_axis',(-0.433012701892223,0.866025403784436,-0.250000000000002));
#2862=DIRECTION('ref_axis',(-0.894427190999914,-0.447213595499962,0.));
#2863=DIRECTION('center_axis',(-0.433012701892223,0.866025403784436,-0.250000000000002));
#2864=DIRECTION('ref_axis',(-0.894427190999914,-0.447213595499962,0.));
#2865=DIRECTION('',(0.433012701892223,-0.866025403784437,0.250000000000002));
#2866=DIRECTION('center_axis',(0.612372435695796,-0.707106781186546,0.353553390593275));
#2867=DIRECTION('ref_axis',(0.5,0.,-0.866025403784438));
#2868=DIRECTION('center_axis',(0.612372435695796,-0.707106781186546,0.353553390593275));
#2869=DIRECTION('ref_axis',(0.755928946018453,0.654653670707979,0.));
#2870=DIRECTION('center_axis',(-0.612372435695796,0.707106781186546,-0.353553390593275));
#2871=DIRECTION('ref_axis',(-0.755928946018453,-0.654653670707979,0.));
#2872=DIRECTION('center_axis',(-0.612372435695796,0.707106781186546,-0.353553390593275));
#2873=DIRECTION('ref_axis',(-0.755928946018453,-0.654653670707979,0.));
#2874=DIRECTION('',(0.612372435695796,-0.707106781186546,0.353553390593275));
#2875=DIRECTION('center_axis',(0.,1.,0.));
#2876=DIRECTION('ref_axis',(0.,0.,1.));
#2877=DIRECTION('center_axis',(0.,1.,0.));
#2878=DIRECTION('ref_axis',(0.,0.,1.));
#2879=DIRECTION('center_axis',(0.,1.,0.));
#2880=DIRECTION('ref_axis',(0.,0.,1.));
#2881=DIRECTION('center_axis',(0.,1.,0.));
#2882=DIRECTION('ref_axis',(0.,0.,1.));
#2883=DIRECTION('',(0.,1.,0.));
#2884=DIRECTION('center_axis',(-0.224143868042018,0.965925826289067,-0.129409522551263));
#2885=DIRECTION('ref_axis',(0.,0.132788176096111,0.991144439670156));
#2886=DIRECTION('center_axis',(-0.224143868042018,0.965925826289067,-0.129409522551263));
#2887=DIRECTION('ref_axis',(-0.974116947696296,-0.22604462437946,0.));
#2888=DIRECTION('center_axis',(-0.224143868042018,0.965925826289067,-0.129409522551263));
#2889=DIRECTION('ref_axis',(-0.974116947696296,-0.22604462437946,0.));
#2890=DIRECTION('center_axis',(-0.224143868042018,0.965925826289067,-0.129409522551263));
#2891=DIRECTION('ref_axis',(-0.974116947696296,-0.22604462437946,0.));
#2892=DIRECTION('',(-0.224143868042018,0.965925826289067,-0.129409522551263));
#2893=DIRECTION('center_axis',(-0.433012701892223,0.866025403784436,-0.250000000000002));
#2894=DIRECTION('ref_axis',(-0.499999999999999,0.,0.866025403784439));
#2895=DIRECTION('center_axis',(-0.433012701892223,0.866025403784436,-0.250000000000002));
#2896=DIRECTION('ref_axis',(-0.894427190999914,-0.447213595499962,0.));
#2897=DIRECTION('center_axis',(-0.433012701892223,0.866025403784436,-0.250000000000002));
#2898=DIRECTION('ref_axis',(-0.894427190999914,-0.447213595499962,0.));
#2899=DIRECTION('center_axis',(-0.433012701892223,0.866025403784436,-0.250000000000002));
#2900=DIRECTION('ref_axis',(-0.894427190999914,-0.447213595499962,0.));
#2901=DIRECTION('',(-0.433012701892223,0.866025403784436,-0.250000000000002));
#2902=DIRECTION('center_axis',(0.866025403784443,0.,0.499999999999992));
#2903=DIRECTION('ref_axis',(0.499999999999992,0.,-0.866025403784443));
#2904=DIRECTION('center_axis',(-0.866025403784443,0.,-0.499999999999992));
#2905=DIRECTION('ref_axis',(-0.499999999999992,0.,0.866025403784443));
#2906=DIRECTION('',(0.866025403784443,0.,0.499999999999992));
#2907=DIRECTION('center_axis',(-0.866025403784443,0.,-0.499999999999992));
#2908=DIRECTION('ref_axis',(-0.499999999999992,0.,0.866025403784443));
#2909=DIRECTION('center_axis',(-0.612372435695796,0.707106781186546,-0.353553390593275));
#2910=DIRECTION('ref_axis',(-0.5,0.,0.866025403784438));
#2911=DIRECTION('center_axis',(-0.612372435695796,0.707106781186546,-0.353553390593275));
#2912=DIRECTION('ref_axis',(-0.755928946018453,-0.654653670707979,0.));
#2913=DIRECTION('center_axis',(-0.612372435695796,0.707106781186546,-0.353553390593275));
#2914=DIRECTION('ref_axis',(-0.755928946018453,-0.654653670707979,0.));
#2915=DIRECTION('center_axis',(-0.612372435695796,0.707106781186546,-0.353553390593275));
#2916=DIRECTION('ref_axis',(-0.755928946018453,-0.654653670707979,0.));
#2917=DIRECTION('',(-0.612372435695796,0.707106781186546,-0.353553390593275));
#2918=DIRECTION('center_axis',(0.,1.,0.));
#2919=DIRECTION('ref_axis',(0.,0.,1.));
#2920=DIRECTION('',(0.,1.,0.));
#2921=DIRECTION('center_axis',(-0.224143868042018,0.965925826289067,-0.129409522551263));
#2922=DIRECTION('ref_axis',(-0.974116947696296,-0.22604462437946,0.));
#2923=DIRECTION('',(-0.224143868042018,0.965925826289067,-0.129409522551263));
#2924=DIRECTION('center_axis',(-0.433012701892223,0.866025403784437,-0.250000000000002));
#2925=DIRECTION('ref_axis',(-0.894427190999914,-0.447213595499962,0.));
#2926=DIRECTION('',(-0.433012701892223,0.866025403784436,-0.250000000000002));
#2927=DIRECTION('center_axis',(-0.612372435695796,0.707106781186546,-0.353553390593275));
#2928=DIRECTION('ref_axis',(-0.755928946018453,-0.654653670707979,0.));
#2929=DIRECTION('',(-0.612372435695796,0.707106781186546,-0.353553390593275));
#2930=DIRECTION('center_axis',(0.433012701892215,0.499999999999992,-0.750000000000008));
#2931=DIRECTION('ref_axis',(-0.866025403784443,0.,-0.499999999999992));
#2932=DIRECTION('center_axis',(0.433012701892215,0.499999999999992,-0.750000000000008));
#2933=DIRECTION('ref_axis',(-0.649519052838319,0.750000000000008,0.125000000000006));
#2934=DIRECTION('center_axis',(-0.433012701892215,-0.499999999999992,0.750000000000008));
#2935=DIRECTION('ref_axis',(0.649519052838319,-0.750000000000008,-0.125000000000006));
#2936=DIRECTION('center_axis',(-0.433012701892215,-0.499999999999992,0.750000000000008));
#2937=DIRECTION('ref_axis',(0.649519052838319,-0.750000000000008,-0.125000000000006));
#2938=DIRECTION('',(0.433012701892215,0.499999999999992,-0.750000000000008));
#2939=DIRECTION('',(-0.433012701892199,-0.500000000000005,0.750000000000008));
#2940=DIRECTION('',(-0.433012701892214,-0.499999999999978,0.750000000000018));
#2941=DIRECTION('center_axis',(-0.433012701892211,0.500000000000004,0.750000000000002));
#2942=DIRECTION('ref_axis',(0.866025403784443,0.,0.499999999999992));
#2943=DIRECTION('center_axis',(-0.433012701892211,0.500000000000004,0.750000000000002));
#2944=DIRECTION('ref_axis',(-0.649519052838324,-0.750000000000002,0.125000000000015));
#2945=DIRECTION('center_axis',(0.433012701892211,-0.500000000000004,-0.750000000000002));
#2946=DIRECTION('ref_axis',(0.649519052838324,0.750000000000002,-0.125000000000015));
#2947=DIRECTION('center_axis',(0.433012701892211,-0.500000000000004,-0.750000000000002));
#2948=DIRECTION('ref_axis',(0.649519052838324,0.750000000000002,-0.125000000000015));
#2949=DIRECTION('',(-0.433012701892211,0.500000000000004,0.750000000000002));
#2950=DIRECTION('',(0.433012701892208,-0.499999999999987,-0.750000000000015));
#2951=DIRECTION('',(0.433012701892233,-0.50000000000002,-0.749999999999979));
#2952=DIRECTION('center_axis',(0.642402019910919,0.482962913144524,-0.595034847165548));
#2953=DIRECTION('ref_axis',(-0.679542161318994,0.,-0.733636456966194));
#2954=DIRECTION('center_axis',(0.642402019910919,0.482962913144524,-0.595034847165548));
#2955=DIRECTION('ref_axis',(0.510942898759438,0.308782699291242,0.802240985506049));
#2956=DIRECTION('center_axis',(-0.642402019910919,-0.482962913144524,0.595034847165548));
#2957=DIRECTION('ref_axis',(-0.510942898759438,-0.308782699291242,-0.802240985506049));
#2958=DIRECTION('center_axis',(-0.642402019910919,-0.482962913144524,0.595034847165548));
#2959=DIRECTION('ref_axis',(-0.510942898759438,-0.308782699291242,-0.802240985506049));
#2960=DIRECTION('',(0.642402019910919,0.482962913144524,-0.595034847165548));
#2961=DIRECTION('center_axis',(-0.194114283826876,0.482962913144539,0.853853892268062));
#2962=DIRECTION('ref_axis',(0.975118889534635,0.,0.221682546161714));
#2963=DIRECTION('center_axis',(-0.194114283826876,0.482962913144539,0.853853892268062));
#2964=DIRECTION('ref_axis',(0.706703285860956,-0.534827323670698,0.463174048936862));
#2965=DIRECTION('center_axis',(0.194114283826876,-0.482962913144539,-0.853853892268062));
#2966=DIRECTION('ref_axis',(-0.706703285860956,0.534827323670698,-0.463174048936862));
#2967=DIRECTION('center_axis',(0.194114283826876,-0.482962913144539,-0.853853892268062));
#2968=DIRECTION('ref_axis',(-0.706703285860956,0.534827323670698,-0.463174048936862));
#2969=DIRECTION('',(-0.194114283826876,0.482962913144539,0.853853892268062));
#2970=DIRECTION('center_axis',(0.808012701892221,0.433012701892207,-0.399519052838338));
#2971=DIRECTION('ref_axis',(-0.443226594010285,0.,-0.89640960858418));
#2972=DIRECTION('center_axis',(0.808012701892221,0.433012701892207,-0.399519052838338));
#2973=DIRECTION('ref_axis',(0.365367827064589,0.163691536870759,0.916357698556077));
#2974=DIRECTION('center_axis',(-0.808012701892221,-0.433012701892208,0.399519052838338));
#2975=DIRECTION('ref_axis',(-0.365367827064589,-0.163691536870759,-0.916357698556077));
#2976=DIRECTION('center_axis',(-0.808012701892221,-0.433012701892207,0.399519052838338));
#2977=DIRECTION('ref_axis',(-0.365367827064589,-0.163691536870759,-0.916357698556077));
#2978=DIRECTION('',(0.808012701892221,0.433012701892207,-0.399519052838338));
#2979=DIRECTION('center_axis',(0.058012701892234,0.433012701892226,0.899519052838325));
#2980=DIRECTION('ref_axis',(0.997926790235505,0.,-0.064359314246356));
#2981=DIRECTION('center_axis',(0.058012701892234,0.433012701892226,0.899519052838325));
#2982=DIRECTION('ref_axis',(0.752666161685325,-0.610905132370716,0.245537305306135));
#2983=DIRECTION('center_axis',(-0.0580127018922341,-0.433012701892225,-0.899519052838325));
#2984=DIRECTION('ref_axis',(-0.752666161685325,0.610905132370716,-0.245537305306135));
#2985=DIRECTION('center_axis',(-0.058012701892234,-0.433012701892226,-0.899519052838325));
#2986=DIRECTION('ref_axis',(-0.752666161685325,0.610905132370716,-0.245537305306135));
#2987=DIRECTION('',(0.058012701892234,0.433012701892226,0.899519052838325));
#2988=DIRECTION('center_axis',(0.918558653543694,0.353553390593261,-0.176776695296649));
#2989=DIRECTION('ref_axis',(-0.188982236504625,0.,-0.981980506061963));
#2990=DIRECTION('center_axis',(0.918558653543694,0.353553390593261,-0.176776695296649));
#2991=DIRECTION('ref_axis',(0.188982236504626,0.,0.981980506061964));
#2992=DIRECTION('center_axis',(-0.918558653543694,-0.353553390593261,0.176776695296649));
#2993=DIRECTION('ref_axis',(-0.188982236504626,-5.55111512312578E-17,-0.981980506061963));
#2994=DIRECTION('center_axis',(-0.918558653543694,-0.353553390593261,0.176776695296649));
#2995=DIRECTION('ref_axis',(-0.188982236504626,0.,-0.981980506061964));
#2996=DIRECTION('',(0.918558653543694,0.353553390593261,-0.176776695296649));
#2997=DIRECTION('center_axis',(0.30618621784791,0.353553390593282,0.883883476483177));
#2998=DIRECTION('ref_axis',(0.944911182523063,0.,-0.327326835354004));
#2999=DIRECTION('center_axis',(0.30618621784791,0.353553390593282,0.883883476483177));
#3000=DIRECTION('ref_axis',(0.755928946018457,-0.654653670707974,-7.66053886991358E-15));
#3001=DIRECTION('center_axis',(-0.30618621784791,-0.353553390593282,-0.883883476483177));
#3002=DIRECTION('ref_axis',(-0.755928946018457,0.654653670707974,7.60502771868232E-15));
#3003=DIRECTION('center_axis',(-0.30618621784791,-0.353553390593282,-0.883883476483177));
#3004=DIRECTION('ref_axis',(-0.755928946018457,0.654653670707974,7.66053886991358E-15));
#3005=DIRECTION('',(0.30618621784791,0.353553390593282,0.883883476483177));
#3006=DIRECTION('center_axis',(0.433012701892215,-0.499999999999992,-0.750000000000008));
#3007=DIRECTION('ref_axis',(0.649519052838319,0.750000000000008,-0.125000000000006));
#3008=DIRECTION('',(0.433012701892215,-0.499999999999992,-0.750000000000008));
#3009=DIRECTION('center_axis',(0.433012701892211,-0.500000000000004,-0.750000000000002));
#3010=DIRECTION('ref_axis',(0.,0.832050294337842,-0.554700196225231));
#3011=DIRECTION('center_axis',(-0.433012701892211,-0.500000000000004,0.750000000000002));
#3012=DIRECTION('ref_axis',(0.649519052838324,-0.750000000000002,-0.125000000000015));
#3013=DIRECTION('',(-0.433012701892211,-0.500000000000004,0.750000000000002));
#3014=DIRECTION('center_axis',(-0.433012701892215,-0.499999999999992,0.750000000000008));
#3015=DIRECTION('ref_axis',(0.,-0.832050294337851,-0.554700196225219));
#3016=DIRECTION('center_axis',(0.194114283826879,-0.482962913144528,-0.853853892268068));
#3017=DIRECTION('ref_axis',(-0.70670328586096,0.534827323670699,-0.463174048936855));
#3018=DIRECTION('',(0.194114283826879,-0.482962913144527,-0.853853892268068));
#3019=DIRECTION('center_axis',(0.194114283826876,-0.482962913144539,-0.853853892268062));
#3020=DIRECTION('ref_axis',(0.,0.87041002959648,-0.492327513326093));
#3021=DIRECTION('center_axis',(-0.642402019910915,-0.482962913144535,0.595034847165542));
#3022=DIRECTION('ref_axis',(-0.510942898759436,-0.308782699291236,-0.802240985506053));
#3023=DIRECTION('',(-0.642402019910915,-0.482962913144535,0.595034847165542));
#3024=DIRECTION('center_axis',(-0.642402019910919,-0.482962913144524,0.595034847165548));
#3025=DIRECTION('ref_axis',(0.679542161318994,0.,0.733636456966194));
#3026=DIRECTION('center_axis',(-0.0580127018922311,-0.433012701892215,-0.89951905283833));
#3027=DIRECTION('ref_axis',(-0.752666161685329,0.610905132370714,-0.245537305306127));
#3028=DIRECTION('',(-0.0580127018922311,-0.433012701892215,-0.89951905283833));
#3029=DIRECTION('center_axis',(-0.0580127018922341,-0.433012701892225,-0.899519052838325));
#3030=DIRECTION('ref_axis',(0.,0.901036538010451,-0.433743192649915));
#3031=DIRECTION('center_axis',(-0.808012701892218,-0.433012701892218,0.399519052838333));
#3032=DIRECTION('ref_axis',(-0.365367827064587,-0.163691536870751,-0.916357698556079));
#3033=DIRECTION('',(-0.808012701892218,-0.433012701892218,0.399519052838333));
#3034=DIRECTION('center_axis',(-0.808012701892221,-0.433012701892208,0.399519052838338));
#3035=DIRECTION('ref_axis',(0.472347490483135,-0.881412416655384,0.));
#3036=DIRECTION('center_axis',(-0.306186217847908,-0.353553390593273,-0.883883476483181));
#3037=DIRECTION('ref_axis',(-0.755928946018462,0.654653670707968,1.58761892521397E-14));
#3038=DIRECTION('',(-0.306186217847908,-0.353553390593273,-0.883883476483181));
#3039=DIRECTION('center_axis',(-0.30618621784791,-0.353553390593282,-0.883883476483177));
#3040=DIRECTION('ref_axis',(0.,0.928476690885255,-0.371390676354114));
#3041=DIRECTION('center_axis',(-0.918558653543692,-0.35355339059327,0.176776695296645));
#3042=DIRECTION('ref_axis',(-0.188982236504625,1.0547118733939E-14,-0.981980506061964));
#3043=DIRECTION('',(-0.918558653543692,-0.35355339059327,0.176776695296645));
#3044=DIRECTION('center_axis',(-0.918558653543694,-0.353553390593261,0.176776695296649));
#3045=DIRECTION('ref_axis',(0.359210604053538,-0.933256525257387,0.));
#3046=DIRECTION('center_axis',(-0.433012701892215,-0.499999999999992,0.750000000000008));
#3047=DIRECTION('ref_axis',(0.866025403784443,0.,0.499999999999992));
#3048=DIRECTION('center_axis',(-0.433012701892215,-0.499999999999992,0.750000000000008));
#3049=DIRECTION('ref_axis',(0.649519052838319,-0.750000000000008,-0.125000000000006));
#3050=DIRECTION('center_axis',(-0.433012701892215,-0.499999999999992,0.750000000000008));
#3051=DIRECTION('ref_axis',(0.649519052838319,-0.750000000000008,-0.125000000000006));
#3052=DIRECTION('',(-0.433012701892215,-0.499999999999992,0.750000000000008));
#3053=DIRECTION('center_axis',(0.433012701892211,-0.500000000000004,-0.750000000000002));
#3054=DIRECTION('ref_axis',(-0.866025403784443,0.,-0.499999999999992));
#3055=DIRECTION('center_axis',(0.433012701892211,-0.500000000000004,-0.750000000000002));
#3056=DIRECTION('ref_axis',(0.649519052838324,0.750000000000002,-0.125000000000015));
#3057=DIRECTION('center_axis',(0.433012701892211,-0.500000000000004,-0.750000000000002));
#3058=DIRECTION('ref_axis',(0.649519052838324,0.750000000000002,-0.125000000000015));
#3059=DIRECTION('',(0.433012701892211,-0.500000000000004,-0.750000000000002));
#3060=DIRECTION('center_axis',(-0.642402019910919,-0.482962913144524,0.595034847165548));
#3061=DIRECTION('ref_axis',(0.679542161318994,0.,0.733636456966194));
#3062=DIRECTION('center_axis',(-0.642402019910919,-0.482962913144524,0.595034847165548));
#3063=DIRECTION('ref_axis',(-0.510942898759438,-0.308782699291242,-0.802240985506049));
#3064=DIRECTION('center_axis',(-0.642402019910919,-0.482962913144524,0.595034847165548));
#3065=DIRECTION('ref_axis',(-0.510942898759438,-0.308782699291242,-0.802240985506049));
#3066=DIRECTION('',(-0.642402019910919,-0.482962913144524,0.595034847165548));
#3067=DIRECTION('center_axis',(0.194114283826876,-0.482962913144539,-0.853853892268062));
#3068=DIRECTION('ref_axis',(-0.975118889534635,0.,-0.221682546161714));
#3069=DIRECTION('center_axis',(0.194114283826876,-0.482962913144539,-0.853853892268062));
#3070=DIRECTION('ref_axis',(-0.706703285860956,0.534827323670698,-0.463174048936862));
#3071=DIRECTION('center_axis',(0.194114283826876,-0.482962913144539,-0.853853892268062));
#3072=DIRECTION('ref_axis',(-0.706703285860956,0.534827323670698,-0.463174048936862));
#3073=DIRECTION('',(0.194114283826876,-0.482962913144539,-0.853853892268062));
#3074=DIRECTION('center_axis',(-0.808012701892221,-0.433012701892208,0.399519052838338));
#3075=DIRECTION('ref_axis',(0.443226594010285,0.,0.89640960858418));
#3076=DIRECTION('center_axis',(-0.808012701892221,-0.433012701892208,0.399519052838338));
#3077=DIRECTION('ref_axis',(-0.365367827064589,-0.163691536870759,-0.916357698556077));
#3078=DIRECTION('center_axis',(-0.808012701892221,-0.433012701892207,0.399519052838338));
#3079=DIRECTION('ref_axis',(-0.365367827064589,-0.163691536870759,-0.916357698556077));
#3080=DIRECTION('',(-0.808012701892221,-0.433012701892207,0.399519052838338));
#3081=DIRECTION('center_axis',(-0.0580127018922341,-0.433012701892225,-0.899519052838325));
#3082=DIRECTION('ref_axis',(-0.997926790235505,0.,0.0643593142463562));
#3083=DIRECTION('center_axis',(-0.0580127018922341,-0.433012701892225,-0.899519052838325));
#3084=DIRECTION('ref_axis',(-0.752666161685325,0.610905132370716,-0.245537305306135));
#3085=DIRECTION('center_axis',(-0.0580127018922342,-0.433012701892225,-0.899519052838325));
#3086=DIRECTION('ref_axis',(-0.752666161685325,0.610905132370716,-0.245537305306135));
#3087=DIRECTION('',(-0.0580127018922342,-0.433012701892225,-0.899519052838325));
#3088=DIRECTION('center_axis',(-0.918558653543694,-0.353553390593261,0.176776695296649));
#3089=DIRECTION('ref_axis',(0.188982236504625,0.,0.981980506061963));
#3090=DIRECTION('center_axis',(-0.918558653543694,-0.353553390593261,0.176776695296649));
#3091=DIRECTION('ref_axis',(-0.188982236504626,-5.55111512312578E-17,-0.981980506061963));
#3092=DIRECTION('center_axis',(-0.918558653543694,-0.353553390593261,0.176776695296649));
#3093=DIRECTION('ref_axis',(-0.188982236504626,0.,-0.981980506061963));
#3094=DIRECTION('',(-0.918558653543694,-0.353553390593261,0.176776695296649));
#3095=DIRECTION('center_axis',(-0.30618621784791,-0.353553390593282,-0.883883476483177));
#3096=DIRECTION('ref_axis',(-0.944911182523063,0.,0.327326835354004));
#3097=DIRECTION('center_axis',(-0.30618621784791,-0.353553390593282,-0.883883476483177));
#3098=DIRECTION('ref_axis',(-0.755928946018457,0.654653670707974,7.60502771868232E-15));
#3099=DIRECTION('center_axis',(-0.306186217847911,-0.353553390593282,-0.883883476483177));
#3100=DIRECTION('ref_axis',(-0.755928946018457,0.654653670707974,7.66053886991358E-15));
#3101=DIRECTION('',(-0.30618621784791,-0.353553390593282,-0.883883476483177));
#3102=DIRECTION('center_axis',(-0.499999999999992,0.,0.866025403784443));
#3103=DIRECTION('ref_axis',(0.866025403784443,0.,0.499999999999992));
#3104=DIRECTION('',(0.866025403784443,0.,0.499999999999992));
#3105=DIRECTION('center_axis',(0.499999999999992,0.,-0.866025403784443));
#3106=DIRECTION('ref_axis',(-0.866025403784443,0.,-0.499999999999992));
#3107=DIRECTION('',(0.866025403784443,0.,0.499999999999992));
#3108=DIRECTION('center_axis',(-0.499999999999999,0.,0.866025403784439));
#3109=DIRECTION('ref_axis',(0.866025403784439,0.,0.499999999999999));
#3110=DIRECTION('',(0.,1.,0.));
#3111=DIRECTION('',(0.866025403784443,0.,0.499999999999992));
#3112=DIRECTION('center_axis',(0.499999999999999,0.,-0.866025403784439));
#3113=DIRECTION('ref_axis',(-0.866025403784439,0.,-0.499999999999999));
#3114=DIRECTION('',(0.866025403784443,0.,0.499999999999992));
#3115=DIRECTION('',(0.,1.,0.));
#3116=DIRECTION('center_axis',(0.866025403784443,0.,0.499999999999992));
#3117=DIRECTION('ref_axis',(0.499999999999992,0.,-0.866025403784443));
#3118=DIRECTION('center_axis',(0.249999999999998,0.866025403784436,-0.433012701892225));
#3119=DIRECTION('ref_axis',(-0.866025403784443,0.,-0.499999999999992));
#3120=DIRECTION('',(0.866025403784443,0.,0.499999999999992));
#3121=DIRECTION('center_axis',(-0.249999999999998,-0.866025403784436,0.433012701892225));
#3122=DIRECTION('ref_axis',(0.866025403784444,0.,0.499999999999991));
#3123=DIRECTION('',(0.866025403784443,0.,0.499999999999992));
#3124=DIRECTION('center_axis',(0.249999999999991,0.866025403784436,-0.433012701892229));
#3125=DIRECTION('ref_axis',(-0.866025403784452,0.,-0.499999999999977));
#3126=DIRECTION('',(0.433012701892214,-0.500000000000001,-0.750000000000002));
#3127=DIRECTION('',(0.866025403784443,0.,0.499999999999992));
#3128=DIRECTION('center_axis',(-0.249999999999991,-0.866025403784436,0.433012701892229));
#3129=DIRECTION('ref_axis',(0.866025403784451,0.,0.499999999999978));
#3130=DIRECTION('',(0.866025403784443,0.,0.499999999999992));
#3131=DIRECTION('',(0.433012701892241,-0.499999999999971,-0.750000000000007));
#3132=DIRECTION('center_axis',(0.866025403784443,0.,0.499999999999992));
#3133=DIRECTION('ref_axis',(0.499999999999992,0.,-0.866025403784443));
#3134=DIRECTION('center_axis',(0.249999999999992,-0.866025403784443,-0.433012701892215));
#3135=DIRECTION('ref_axis',(0.,0.447213595499952,-0.894427190999919));
#3136=DIRECTION('',(0.866025403784443,0.,0.499999999999992));
#3137=DIRECTION('center_axis',(-0.249999999999991,0.866025403784443,0.433012701892215));
#3138=DIRECTION('ref_axis',(0.,-0.447213595499952,0.894427190999919));
#3139=DIRECTION('',(0.866025403784443,0.,0.499999999999992));
#3140=DIRECTION('center_axis',(0.249999999999984,-0.866025403784443,-0.433012701892219));
#3141=DIRECTION('ref_axis',(0.,0.447213595499956,-0.894427190999917));
#3142=DIRECTION('',(-0.433012701892197,-0.499999999999982,0.750000000000025));
#3143=DIRECTION('',(0.866025403784443,0.,0.499999999999992));
#3144=DIRECTION('center_axis',(-0.249999999999985,0.866025403784443,0.433012701892219));
#3145=DIRECTION('ref_axis',(0.,-0.447213595499956,0.894427190999917));
#3146=DIRECTION('',(0.866025403784443,0.,0.499999999999992));
#3147=DIRECTION('',(-0.433012701892228,-0.49999999999999,0.750000000000002));
#3148=DIRECTION('center_axis',(0.866025403784443,0.,0.499999999999992));
#3149=DIRECTION('ref_axis',(0.499999999999992,0.,-0.866025403784443));
#3150=DIRECTION('center_axis',(-0.499999999999992,0.,0.866025403784443));
#3151=DIRECTION('ref_axis',(0.866025403784443,0.,0.499999999999992));
#3152=DIRECTION('',(0.866025403784442,0.,0.499999999999994));
#3153=DIRECTION('center_axis',(0.499999999999992,0.,-0.866025403784443));
#3154=DIRECTION('ref_axis',(-0.866025403784443,0.,-0.499999999999992));
#3155=DIRECTION('',(0.866025403784443,0.,0.499999999999992));
#3156=DIRECTION('center_axis',(0.,1.,0.));
#3157=DIRECTION('ref_axis',(0.,0.,1.));
#3158=DIRECTION('center_axis',(0.249999999999992,-0.866025403784443,-0.433012701892215));
#3159=DIRECTION('ref_axis',(0.,0.447213595499952,-0.894427190999919));
#3160=DIRECTION('',(0.866025403784443,0.,0.499999999999992));
#3161=DIRECTION('center_axis',(-0.249999999999992,0.866025403784443,0.433012701892215));
#3162=DIRECTION('ref_axis',(0.,-0.447213595499952,0.894427190999919));
#3163=DIRECTION('',(0.866025403784444,0.,0.499999999999991));
#3164=DIRECTION('center_axis',(-0.433012701892215,-0.499999999999992,0.750000000000008));
#3165=DIRECTION('ref_axis',(0.866025403784443,0.,0.499999999999992));
#3166=DIRECTION('center_axis',(0.249999999999998,0.866025403784436,-0.433012701892225));
#3167=DIRECTION('ref_axis',(-0.866025403784443,0.,-0.499999999999992));
#3168=DIRECTION('',(0.866025403784442,0.,0.499999999999994));
#3169=DIRECTION('center_axis',(-0.249999999999998,-0.866025403784436,0.433012701892225));
#3170=DIRECTION('ref_axis',(0.866025403784443,0.,0.499999999999992));
#3171=DIRECTION('',(0.866025403784442,0.,0.499999999999994));
#3172=DIRECTION('center_axis',(0.433012701892211,-0.500000000000004,-0.750000000000002));
#3173=DIRECTION('ref_axis',(-0.866025403784443,0.,-0.499999999999992));
#3337=CARTESIAN_POINT('',(0.,0.,0.));
#3338=CARTESIAN_POINT('Origin',(-69.7150450046476,109.,-52.2499999999992));
#3339=CARTESIAN_POINT('',(-57.0362860918569,101.937180526611,-60.2102546138697));
#3340=CARTESIAN_POINT('',(-60.5003877069947,101.937180526611,-62.2102546138697));
#3341=CARTESIAN_POINT('',(-60.5003877069947,101.937180526611,-62.2102546138697));
#3342=CARTESIAN_POINT('',(-63.4028671781572,123.991664350565,-49.1830127018903));
#3343=CARTESIAN_POINT('Origin',(-63.6528671781565,109.,-48.7499999999993));
#3344=CARTESIAN_POINT('',(-66.866968793295,123.991664350565,-51.1830127018903));
#3345=CARTESIAN_POINT('',(-66.866968793295,123.991664350565,-51.1830127018903));
#3346=CARTESIAN_POINT('Origin',(-67.1169687932943,109.,-50.7499999999993));
#3347=CARTESIAN_POINT('Origin',(-69.7150450046476,109.,-52.2499999999992));
#3348=CARTESIAN_POINT('',(-60.7503877069946,101.071155122826,-61.7772419119775));
#3349=CARTESIAN_POINT('',(-57.2862860918569,101.071155122826,-59.7772419119775));
#3350=CARTESIAN_POINT('',(-60.7503877069946,101.071155122826,-61.7772419119775));
#3351=CARTESIAN_POINT('',(-73.4835498795932,101.071155122824,-39.7227580880222));
#3352=CARTESIAN_POINT('Origin',(-67.1169687932943,109.,-50.7499999999993));
#3353=CARTESIAN_POINT('',(-70.0194482644555,101.071155122824,-37.7227580880222));
#3354=CARTESIAN_POINT('',(-73.4835498795932,101.071155122824,-39.7227580880221));
#3355=CARTESIAN_POINT('Origin',(-63.6528671781565,109.,-48.7499999999993));
#3356=CARTESIAN_POINT('Origin',(-119.078493020361,109.,-80.7499999999988));
#3357=CARTESIAN_POINT('',(-65.5747753124034,96.49269543419,-59.421157464004));
#3358=CARTESIAN_POINT('',(-73.855314696892,96.4926954341901,-45.0788425359943));
#3359=CARTESIAN_POINT('Origin',(-69.7150450046476,109.,-52.2499999999992));
#3360=CARTESIAN_POINT('',(-123.218762712605,96.4926954341901,-73.5788425359939));
#3361=CARTESIAN_POINT('',(-123.218762712605,96.4926954341901,-73.5788425359939));
#3362=CARTESIAN_POINT('',(-114.938223328117,96.49269543419,-87.9211574640035));
#3363=CARTESIAN_POINT('Origin',(-119.078493020361,109.,-80.7499999999988));
#3364=CARTESIAN_POINT('',(-114.938223328117,96.49269543419,-87.9211574640035));
#3365=CARTESIAN_POINT('Origin',(-119.078493020361,109.,-80.7499999999988));
#3366=CARTESIAN_POINT('',(-94.3860089394201,105.235685467736,-49.7275542973482));
#3367=CARTESIAN_POINT('',(-82.8207084929668,105.235685467736,-43.0503249713298));
#3368=CARTESIAN_POINT('',(-94.3860089394201,105.235685467737,-49.7275542973482));
#3369=CARTESIAN_POINT('',(-91.0176401746589,103.250749366077,-48.5513043322017));
#3370=CARTESIAN_POINT('Ctrl Pts',(-91.0176401746589,103.250749366077,-48.5513043322017));
#3371=CARTESIAN_POINT('Ctrl Pts',(-91.2361059276669,103.557750420993,-48.5303294493383));
#3372=CARTESIAN_POINT('Ctrl Pts',(-91.4832335600058,103.842139746856,-48.5508334265686));
#3373=CARTESIAN_POINT('Ctrl Pts',(-92.1066673879442,104.430592760333,-48.6750977465524));
#3374=CARTESIAN_POINT('Ctrl Pts',(-92.5431699718694,104.735168552794,-48.8223964645982));
#3375=CARTESIAN_POINT('Ctrl Pts',(-93.461912716518,105.137985045737,-49.2219363914119));
#3376=CARTESIAN_POINT('Ctrl Pts',(-93.9449426785634,105.235685467736,-49.4729045729122));
#3377=CARTESIAN_POINT('Ctrl Pts',(-94.3860089394201,105.235685467736,-49.7275542973483));
#3378=CARTESIAN_POINT('',(-92.3860089394197,98.3074822374609,-53.1916559124865));
#3379=CARTESIAN_POINT('Ctrl Pts',(-92.3860089394197,98.307482237461,-53.1916559124864));
#3380=CARTESIAN_POINT('Ctrl Pts',(-91.944942678563,98.307482237461,-52.9370061880504));
#3381=CARTESIAN_POINT('Ctrl Pts',(-91.5102607802988,98.3772644212952,-52.6022967036335));
#3382=CARTESIAN_POINT('Ctrl Pts',(-90.7942826050959,98.676845000861,-51.8515582405649));
#3383=CARTESIAN_POINT('Ctrl Pts',(-90.5123369230427,98.9076700218055,-51.4365591158164));
#3384=CARTESIAN_POINT('Ctrl Pts',(-90.1413389560881,99.4578375470661,-50.6726253387866));
#3385=CARTESIAN_POINT('Ctrl Pts',(-90.0255053791506,99.8112989429842,-50.2740223286365));
#3386=CARTESIAN_POINT('Ctrl Pts',(-89.9729277960154,100.614428273412,-49.573341944019));
#3387=CARTESIAN_POINT('Ctrl Pts',(-90.0353007740436,101.064744995698,-49.2720751413297));
#3388=CARTESIAN_POINT('Ctrl Pts',(-90.2865953679429,101.9352550043,-48.8368201370289));
#3389=CARTESIAN_POINT('Ctrl Pts',(-90.4922380489042,102.413371759201,-48.6738702011243));
#3390=CARTESIAN_POINT('Ctrl Pts',(-90.8440070426079,102.99654996933,-48.5751774684912));
#3391=CARTESIAN_POINT('Ctrl Pts',(-90.9285040512729,103.125489990024,-48.559862285662));
#3392=CARTESIAN_POINT('Ctrl Pts',(-91.0176401746589,103.250749366077,-48.5513043322017));
#3393=CARTESIAN_POINT('',(-80.8207084929665,98.3074822374608,-46.5144265864682));
#3394=CARTESIAN_POINT('',(-92.3860089394198,98.3074822374611,-53.1916559124864));
#3395=CARTESIAN_POINT('',(-84.4784050214276,104.702740240336,-44.1791103605043));
#3396=CARTESIAN_POINT('Ctrl Pts',(-84.4784050214273,104.702740240336,-44.179110360504));
#3397=CARTESIAN_POINT('Ctrl Pts',(-84.719910157753,104.526945752297,-44.3792409314819));
#3398=CARTESIAN_POINT('Ctrl Pts',(-84.9292227283709,104.313493521274,-44.5780840276366));
#3399=CARTESIAN_POINT('Ctrl Pts',(-85.3433081511931,103.743726568118,-45.0453786543482));
#3400=CARTESIAN_POINT('Ctrl Pts',(-85.5286602574863,103.319666529342,-45.3392616445606));
#3401=CARTESIAN_POINT('Ctrl Pts',(-85.6804888744289,102.416155145618,-45.8942563092267));
#3402=CARTESIAN_POINT('Ctrl Pts',(-85.6462202716666,101.937209973523,-46.1563950132377));
#3403=CARTESIAN_POINT('Ctrl Pts',(-85.3937969757602,101.062790026475,-46.5936049867616));
#3404=CARTESIAN_POINT('Ctrl Pts',(-85.1596379659028,100.611874672147,-46.7963965459624));
#3405=CARTESIAN_POINT('Ctrl Pts',(-84.5153961509797,99.8096167014324,-47.0942865585158));
#3406=CARTESIAN_POINT('Ctrl Pts',(-84.1059621410022,99.4574342557325,-47.1885248105415));
#3407=CARTESIAN_POINT('Ctrl Pts',(-83.2575101221815,98.9126166677475,-47.2430172368065));
#3408=CARTESIAN_POINT('Ctrl Pts',(-82.7609372275344,98.6829050367047,-47.2068324926174));
#3409=CARTESIAN_POINT('Ctrl Pts',(-81.7609021788356,98.3807025943171,-46.9694819795316));
#3410=CARTESIAN_POINT('Ctrl Pts',(-81.2579982865691,98.3074822374608,-46.7668959665184));
#3411=CARTESIAN_POINT('Ctrl Pts',(-80.8207084929665,98.3074822374608,-46.5144265864681));
#3412=CARTESIAN_POINT('Ctrl Pts',(-82.8207084929668,105.235685467736,-43.0503249713298));
#3413=CARTESIAN_POINT('Ctrl Pts',(-83.2579982865694,105.235685467736,-43.3027943513801));
#3414=CARTESIAN_POINT('Ctrl Pts',(-83.7101950061769,105.133251025885,-43.5932077637468));
#3415=CARTESIAN_POINT('Ctrl Pts',(-84.2375848518395,104.864030249166,-43.985328869011));
#3416=CARTESIAN_POINT('Ctrl Pts',(-84.3616836412502,104.787703134226,-44.0823856414543));
#3417=CARTESIAN_POINT('Ctrl Pts',(-84.4784050214273,104.702740240336,-44.179110360504));
#3418=CARTESIAN_POINT('Origin',(-119.078493020361,109.,-80.7499999999988));
#3419=CARTESIAN_POINT('',(-105.931810542547,105.235685467737,-56.3935259609235));
#3420=CARTESIAN_POINT('',(-105.931810542547,105.235685467737,-56.3935259609236));
#3421=CARTESIAN_POINT('',(-102.208219994794,103.102717662028,-55.0841964154936));
#3422=CARTESIAN_POINT('Ctrl Pts',(-102.208219994794,103.102717662026,-55.0841964154936));
#3423=CARTESIAN_POINT('Ctrl Pts',(-102.449021592923,103.452288080539,-55.0506293513879));
#3424=CARTESIAN_POINT('Ctrl Pts',(-102.730142130046,103.775612080798,-55.0719387240821));
#3425=CARTESIAN_POINT('Ctrl Pts',(-103.427690853637,104.41668799164,-55.2155771708353));
#3426=CARTESIAN_POINT('Ctrl Pts',(-103.909507673844,104.73291730259,-55.385468864601));
#3427=CARTESIAN_POINT('Ctrl Pts',(-104.920531073176,105.142197830513,-55.8362211929756));
#3428=CARTESIAN_POINT('Ctrl Pts',(-105.450263434612,105.235685467736,-56.1155046085297));
#3429=CARTESIAN_POINT('Ctrl Pts',(-105.931810542547,105.235685467736,-56.3935259609236));
#3430=CARTESIAN_POINT('',(-103.931810542547,98.307482237461,-59.8576275760617));
#3431=CARTESIAN_POINT('Ctrl Pts',(-103.931810542547,98.3074822374611,-59.8576275760617));
#3432=CARTESIAN_POINT('Ctrl Pts',(-103.450263434612,98.3074822374611,-59.5796062236677));
#3433=CARTESIAN_POINT('Ctrl Pts',(-102.966762319561,98.3741443355121,-59.2202479404765));
#3434=CARTESIAN_POINT('Ctrl Pts',(-102.161749770577,98.6785063270139,-58.4126743523891));
#3435=CARTESIAN_POINT('Ctrl Pts',(-101.840308730574,98.9178350152992,-57.9650036590062));
#3436=CARTESIAN_POINT('Ctrl Pts',(-101.440098436538,99.4841271059821,-57.1713087801904));
#3437=CARTESIAN_POINT('Ctrl Pts',(-101.317391802105,99.8312991080725,-56.7758910574572));
#3438=CARTESIAN_POINT('Ctrl Pts',(-101.255012945074,100.623349028226,-56.0804534046886));
#3439=CARTESIAN_POINT('Ctrl Pts',(-101.314116564966,101.068801289505,-55.7811982784879));
#3440=CARTESIAN_POINT('Ctrl Pts',(-101.563069256545,101.931198710494,-55.3499995679935));
#3441=CARTESIAN_POINT('Ctrl Pts',(-101.769030711735,102.403958803925,-55.1901485168392));
#3442=CARTESIAN_POINT('Ctrl Pts',(-102.095779742704,102.93486881927,-55.1031827978842));
#3443=CARTESIAN_POINT('Ctrl Pts',(-102.150902897407,103.019510732018,-55.0921862573272));
#3444=CARTESIAN_POINT('Ctrl Pts',(-102.208219994794,103.102717662026,-55.0841964154936));
#3445=CARTESIAN_POINT('',(-103.931810542547,98.3074822374611,-59.8576275760617));
#3446=CARTESIAN_POINT('Ctrl Pts',(-94.3860089394201,105.235685467736,-49.7275542973483));
#3447=CARTESIAN_POINT('Ctrl Pts',(-94.8437110509037,105.235685467736,-49.991808734622));
#3448=CARTESIAN_POINT('Ctrl Pts',(-95.3183294965658,105.131719766023,-50.2956435885911));
#3449=CARTESIAN_POINT('Ctrl Pts',(-96.1649446403336,104.726122671488,-50.9165050382747));
#3450=CARTESIAN_POINT('Ctrl Pts',(-96.5365223340826,104.425439262705,-51.2347212917227));
#3451=CARTESIAN_POINT('Ctrl Pts',(-97.079067270285,103.751330105903,-51.8179767152385));
#3452=CARTESIAN_POINT('Ctrl Pts',(-97.2914477713889,103.33295780308,-52.124268380383));
#3453=CARTESIAN_POINT('Ctrl Pts',(-97.4838471817179,102.430163538116,-52.7010684635898));
#3454=CARTESIAN_POINT('Ctrl Pts',(-97.4623083504636,101.946025606973,-52.9725395573328));
#3455=CARTESIAN_POINT('Ctrl Pts',(-97.2047953462119,101.053974393026,-53.4185651643064));
#3456=CARTESIAN_POINT('Ctrl Pts',(-96.9552287340129,100.59897551963,-53.616662472833));
#3457=CARTESIAN_POINT('Ctrl Pts',(-96.2710769848093,99.7982897132515,-53.8916024252977));
#3458=CARTESIAN_POINT('Ctrl Pts',(-95.8377694343555,99.451348267594,-53.9679676343933));
#3459=CARTESIAN_POINT('Ctrl Pts',(-94.9448662844064,98.9117809702792,-53.991550437936));
#3460=CARTESIAN_POINT('Ctrl Pts',(-94.4206402272791,98.683674936935,-53.9377289055515));
#3461=CARTESIAN_POINT('Ctrl Pts',(-93.3698028357836,98.3818254132703,-53.670590764968));
#3462=CARTESIAN_POINT('Ctrl Pts',(-92.8437110509033,98.307482237461,-53.4559103497602));
#3463=CARTESIAN_POINT('Ctrl Pts',(-92.3860089394197,98.307482237461,-53.1916559124864));
#3464=CARTESIAN_POINT('Origin',(-119.078493020361,109.,-80.7499999999988));
#3465=CARTESIAN_POINT('',(-117.424340315019,105.235685467737,-63.0287411187298));
#3466=CARTESIAN_POINT('',(-117.424340315019,105.235685467737,-63.0287411187298));
#3467=CARTESIAN_POINT('',(-112.873099678569,102.847499823892,-61.3708278876974));
#3468=CARTESIAN_POINT('Ctrl Pts',(-112.873099678569,102.847499823892,-61.3708278876974));
#3469=CARTESIAN_POINT('Ctrl Pts',(-112.885263071986,102.865530125643,-61.3684870415431));
#3470=CARTESIAN_POINT('Ctrl Pts',(-112.897548248638,102.883504310233,-61.366295141775));
#3471=CARTESIAN_POINT('Ctrl Pts',(-113.223445655223,103.354153784421,-61.312605698808));
#3472=CARTESIAN_POINT('Ctrl Pts',(-113.617943081627,103.765699546249,-61.3609453836262));
#3473=CARTESIAN_POINT('Ctrl Pts',(-114.51341914509,104.46875863804,-61.596335766007));
#3474=CARTESIAN_POINT('Ctrl Pts',(-115.084650741731,104.772419738951,-61.8242044014969));
#3475=CARTESIAN_POINT('Ctrl Pts',(-116.26458534071,105.155153282331,-62.3819677418281));
#3476=CARTESIAN_POINT('Ctrl Pts',(-116.873387883958,105.235685467737,-62.7106485843461));
#3477=CARTESIAN_POINT('Ctrl Pts',(-117.424340315019,105.235685467736,-63.0287411187299));
#3478=CARTESIAN_POINT('',(-115.424340315019,98.3074822374612,-66.4928427338677));
#3479=CARTESIAN_POINT('Ctrl Pts',(-115.424340315019,98.3074822374612,-66.4928427338678));
#3480=CARTESIAN_POINT('Ctrl Pts',(-114.873387883957,98.3074822374612,-66.1747501994839));
#3481=CARTESIAN_POINT('Ctrl Pts',(-114.304395627967,98.3648569324462,-65.7771159167707));
#3482=CARTESIAN_POINT('Ctrl Pts',(-113.316922034078,98.6488278676478,-64.8860003371488));
#3483=CARTESIAN_POINT('Ctrl Pts',(-112.899248494017,98.8771074785532,-64.3921613457507));
#3484=CARTESIAN_POINT('Ctrl Pts',(-112.369176942676,99.4398467473837,-63.5238717830588));
#3485=CARTESIAN_POINT('Ctrl Pts',(-112.191730388089,99.7801872611806,-63.0995889604281));
#3486=CARTESIAN_POINT('Ctrl Pts',(-112.057561335007,100.581884791004,-62.3492963885222));
#3487=CARTESIAN_POINT('Ctrl Pts',(-112.099359165682,101.044133890221,-62.0245059301422));
#3488=CARTESIAN_POINT('Ctrl Pts',(-112.357346552702,101.937828414283,-61.5776586681113));
#3489=CARTESIAN_POINT('Ctrl Pts',(-112.577858013516,102.409850877713,-61.4276471726289));
#3490=CARTESIAN_POINT('Ctrl Pts',(-112.873099678569,102.847499823891,-61.3708278876975));
#3491=CARTESIAN_POINT('',(-115.424340315019,98.3074822374611,-66.4928427338679));
#3492=CARTESIAN_POINT('Ctrl Pts',(-105.931810542547,105.235685467736,-56.3935259609236));
#3493=CARTESIAN_POINT('Ctrl Pts',(-106.441097653729,105.235685467736,-56.687563011659));
#3494=CARTESIAN_POINT('Ctrl Pts',(-106.974640486628,105.132960205187,-57.0250658019486));
#3495=CARTESIAN_POINT('Ctrl Pts',(-107.947581410815,104.730808636537,-57.7176366639949));
#3496=CARTESIAN_POINT('Ctrl Pts',(-108.386686426508,104.432320373104,-58.0736604657704));
#3497=CARTESIAN_POINT('Ctrl Pts',(-109.030432576161,103.765790736202,-58.7123084319066));
#3498=CARTESIAN_POINT('Ctrl Pts',(-109.294438065739,103.359086193815,-59.0420063444297));
#3499=CARTESIAN_POINT('Ctrl Pts',(-109.56709842014,102.458977333711,-59.6612621436709));
#3500=CARTESIAN_POINT('Ctrl Pts',(-109.572926265459,101.965344390994,-59.9517288812603));
#3501=CARTESIAN_POINT('Ctrl Pts',(-109.304259556052,101.034655609004,-60.4170732722551));
#3502=CARTESIAN_POINT('Ctrl Pts',(-109.022522963702,100.572512615502,-60.6044945027757));
#3503=CARTESIAN_POINT('Ctrl Pts',(-108.260113770694,99.7760817327768,-60.8335085749491));
#3504=CARTESIAN_POINT('Ctrl Pts',(-107.781619042588,99.4397737575475,-60.8753169212342));
#3505=CARTESIAN_POINT('Ctrl Pts',(-106.791454021988,98.9062732240887,-60.8366840402783));
#3506=CARTESIAN_POINT('Ctrl Pts',(-106.200906509653,98.6801492903,-60.7429663371135));
#3507=CARTESIAN_POINT('Ctrl Pts',(-105.025500473564,98.3809411378044,-60.40107533564));
#3508=CARTESIAN_POINT('Ctrl Pts',(-104.441097653728,98.3074822374611,-60.1516646267969));
#3509=CARTESIAN_POINT('Ctrl Pts',(-103.931810542547,98.3074822374611,-59.8576275760616));
#3510=CARTESIAN_POINT('Origin',(-119.078493020361,109.,-80.7499999999988));
#3511=CARTESIAN_POINT('',(-118.78998649473,98.3074822374612,-68.4359994617213));
#3512=CARTESIAN_POINT('',(-118.78998649473,98.3074822374611,-68.4359994617214));
#3513=CARTESIAN_POINT('Ctrl Pts',(-117.424340315019,105.235685467736,-63.0287411187299));
#3514=CARTESIAN_POINT('Ctrl Pts',(-118.104455067791,105.235685467737,-63.4214055543222));
#3515=CARTESIAN_POINT('Ctrl Pts',(-118.823383370921,105.115025708115,-63.8707727019096));
#3516=CARTESIAN_POINT('Ctrl Pts',(-120.152211057545,104.638615075121,-64.7952439254207));
#3517=CARTESIAN_POINT('Ctrl Pts',(-120.762708154872,104.285378551405,-65.27078272247));
#3518=CARTESIAN_POINT('Ctrl Pts',(-121.530321038309,103.561110088859,-66.0199577490771));
#3519=CARTESIAN_POINT('Ctrl Pts',(-121.807474740758,103.201357059968,-66.343360523086));
#3520=CARTESIAN_POINT('Ctrl Pts',(-122.043414724861,102.594072465734,-66.7981024939494));
#3521=CARTESIAN_POINT('Ctrl Pts',(-122.092678493038,102.380375656682,-66.945003657385));
#3522=CARTESIAN_POINT('Ctrl Pts',(-122.117297884372,101.943528113597,-67.2175789887018));
#3523=CARTESIAN_POINT('Ctrl Pts',(-122.092529257229,101.720365047742,-67.3432446008741));
#3524=CARTESIAN_POINT('Ctrl Pts',(-121.965301437595,101.279634952257,-67.5636096486164));
#3525=CARTESIAN_POINT('Ctrl Pts',(-121.863134141106,101.063079080039,-67.6578035054809));
#3526=CARTESIAN_POINT('Ctrl Pts',(-121.5934173484,100.650884319169,-67.8097493261416));
#3527=CARTESIAN_POINT('Ctrl Pts',(-121.425973083727,100.45519187943,-67.8675427871017));
#3528=CARTESIAN_POINT('Ctrl Pts',(-120.858109129937,99.9126581141667,-67.9877099959866));
#3529=CARTESIAN_POINT('Ctrl Pts',(-120.389803254753,99.6102405927516,-67.9953924971306));
#3530=CARTESIAN_POINT('Ctrl Pts',(-119.242323386653,99.0186112201875,-67.9041663880787));
#3531=CARTESIAN_POINT('Ctrl Pts',(-118.452225355267,98.7496918581534,-67.7397055339048));
#3532=CARTESIAN_POINT('Ctrl Pts',(-116.883055382911,98.393532390957,-67.231519360489));
#3533=CARTESIAN_POINT('Ctrl Pts',(-116.10445506779,98.3074822374612,-66.8855071694601));
#3534=CARTESIAN_POINT('Ctrl Pts',(-115.424340315019,98.3074822374612,-66.4928427338678));
#3535=CARTESIAN_POINT('',(-120.78998649473,105.235685467737,-64.9718978465832));
#3536=CARTESIAN_POINT('',(-120.78998649473,105.235685467737,-64.9718978465831));
#3537=CARTESIAN_POINT('Ctrl Pts',(-118.78998649473,98.3074822374612,-68.4359994617213));
#3538=CARTESIAN_POINT('Ctrl Pts',(-118.918348276834,98.3074822374612,-68.5101091711724));
#3539=CARTESIAN_POINT('Ctrl Pts',(-119.051966028522,98.319606062948,-68.5729797213706));
#3540=CARTESIAN_POINT('Ctrl Pts',(-119.390180292013,98.3776312711511,-68.7006060360938));
#3541=CARTESIAN_POINT('Ctrl Pts',(-119.594844068455,98.4360499331429,-68.7509667466566));
#3542=CARTESIAN_POINT('Ctrl Pts',(-120.108561068232,98.6351217911646,-68.822841039124));
#3543=CARTESIAN_POINT('Ctrl Pts',(-120.410333239601,98.8023575570841,-68.8132768624661));
#3544=CARTESIAN_POINT('Ctrl Pts',(-121.095658711484,99.2862798538955,-68.7087637376292));
#3545=CARTESIAN_POINT('Ctrl Pts',(-121.453647702316,99.6436546824008,-68.5719722406892));
#3546=CARTESIAN_POINT('Ctrl Pts',(-121.95322023847,100.313709548206,-68.2828712619504));
#3547=CARTESIAN_POINT('Ctrl Pts',(-122.13026373805,100.619480486203,-68.1403943115824));
#3548=CARTESIAN_POINT('Ctrl Pts',(-122.350414930589,101.118875846441,-67.8997101912188));
#3549=CARTESIAN_POINT('Ctrl Pts',(-122.419254299142,101.308117977183,-67.8067240343058));
#3550=CARTESIAN_POINT('Ctrl Pts',(-122.529732701345,101.690626616667,-67.6154765320548));
#3551=CARTESIAN_POINT('Ctrl Pts',(-122.571615353665,101.884694244957,-67.5168156573903));
#3552=CARTESIAN_POINT('Ctrl Pts',(-122.647401154913,102.409372784178,-67.2455011686517));
#3553=CARTESIAN_POINT('Ctrl Pts',(-122.655932486104,102.745023337843,-67.0673187398412));
#3554=CARTESIAN_POINT('Ctrl Pts',(-122.572273917842,103.513663673561,-66.6372167411127));
#3555=CARTESIAN_POINT('Ctrl Pts',(-122.443353045988,103.95119638048,-66.3765548091624));
#3556=CARTESIAN_POINT('Ctrl Pts',(-122.075417244245,104.56927639081,-65.9299074078767));
#3557=CARTESIAN_POINT('Ctrl Pts',(-121.885875205944,104.790787749988,-65.7451136026938));
#3558=CARTESIAN_POINT('Ctrl Pts',(-121.506987477856,105.058995953627,-65.4396037944961));
#3559=CARTESIAN_POINT('Ctrl Pts',(-121.342237738227,105.139116769073,-65.3199491226463));
#3560=CARTESIAN_POINT('Ctrl Pts',(-121.043690674034,105.218909586375,-65.1233635722866));
#3561=CARTESIAN_POINT('Ctrl Pts',(-120.918381560469,105.235685467737,-65.0460267723497));
#3562=CARTESIAN_POINT('Ctrl Pts',(-120.78998649473,105.235685467737,-64.9718978465831));
#3563=CARTESIAN_POINT('Origin',(-119.078493020361,109.,-80.7499999999988));
#3564=CARTESIAN_POINT('',(-66.3693581073396,122.42480974691,-58.0448996923544));
#3565=CARTESIAN_POINT('',(-62.2290884150953,108.0824948189,-65.2160571563592));
#3566=CARTESIAN_POINT('Origin',(-69.7150450046476,109.,-52.2499999999992));
#3567=CARTESIAN_POINT('',(-111.592536430809,108.0824948189,-93.7160571563587));
#3568=CARTESIAN_POINT('',(-111.592536430809,108.0824948189,-93.7160571563587));
#3569=CARTESIAN_POINT('',(-115.732806123053,122.42480974691,-86.5448996923539));
#3570=CARTESIAN_POINT('Origin',(-119.078493020361,109.,-80.7499999999988));
#3571=CARTESIAN_POINT('',(-115.732806123053,122.42480974691,-86.5448996923539));
#3572=CARTESIAN_POINT('Origin',(-119.078493020361,109.,-80.7499999999988));
#3573=CARTESIAN_POINT('',(-81.8660249138711,98.3074822374625,-71.4128027395503));
#3574=CARTESIAN_POINT('',(-70.3007244674178,98.3074822374627,-64.7355734135318));
#3575=CARTESIAN_POINT('',(-81.8660249138712,98.3074822374623,-71.4128027395501));
#3576=CARTESIAN_POINT('',(-78.1372951281693,99.8763092742309,-70.8607163717404));
#3577=CARTESIAN_POINT('Ctrl Pts',(-78.1372951281693,99.8763092742309,-70.8607163717404));
#3578=CARTESIAN_POINT('Ctrl Pts',(-78.3931479940217,99.6124791386442,-70.7749851098822));
#3579=CARTESIAN_POINT('Ctrl Pts',(-78.6840646784847,99.3786530548441,-70.7196442240182));
#3580=CARTESIAN_POINT('Ctrl Pts',(-79.4092304936657,98.9076700218071,-70.6677035733428));
#3581=CARTESIAN_POINT('Ctrl Pts',(-79.9096031192728,98.6768450008626,-70.704376134114));
#3582=CARTESIAN_POINT('Ctrl Pts',(-80.9177507874897,98.3772644212968,-70.9490621908606));
#3583=CARTESIAN_POINT('Ctrl Pts',(-81.4249586530144,98.3074822374626,-71.1581530151143));
#3584=CARTESIAN_POINT('Ctrl Pts',(-81.8660249138711,98.3074822374626,-71.4128027395504));
#3585=CARTESIAN_POINT('',(-79.8660249138713,105.235685467738,-74.8769043546876));
#3586=CARTESIAN_POINT('Ctrl Pts',(-79.8660249138713,105.235685467738,-74.8769043546876));
#3587=CARTESIAN_POINT('Ctrl Pts',(-79.4249586530146,105.235685467738,-74.6222546302515));
#3588=CARTESIAN_POINT('Ctrl Pts',(-78.966098851271,105.13798504574,-74.3294225030814));
#3589=CARTESIAN_POINT('Ctrl Pts',(-78.1607157524998,104.735168552796,-73.7335379100799));
#3590=CARTESIAN_POINT('Ctrl Pts',(-77.8149000287647,104.430592760335,-73.4291649426061));
#3591=CARTESIAN_POINT('Ctrl Pts',(-77.3250662827369,103.743205497,-72.8710607726881));
#3592=CARTESIAN_POINT('Ctrl Pts',(-77.1468233216009,103.317679951548,-72.580553986839));
#3593=CARTESIAN_POINT('Ctrl Pts',(-77.0066222737195,102.413371759203,-72.0316418950969));
#3594=CARTESIAN_POINT('Ctrl Pts',(-77.0449197172773,101.935255004302,-71.7720751413298));
#3595=CARTESIAN_POINT('Ctrl Pts',(-77.2962143111765,101.0647449957,-71.3368201370292));
#3596=CARTESIAN_POINT('Ctrl Pts',(-77.5259325266081,100.614428273414,-71.1321701522025));
#3597=CARTESIAN_POINT('Ctrl Pts',(-77.9342089099037,100.096499176469,-70.9356037497933));
#3598=CARTESIAN_POINT('Ctrl Pts',(-78.0329047040169,99.9839545009761,-70.895695549162));
#3599=CARTESIAN_POINT('Ctrl Pts',(-78.1372951281693,99.8763092742309,-70.8607163717404));
#3600=CARTESIAN_POINT('',(-68.3007244674181,105.235685467739,-68.1996750286692));
#3601=CARTESIAN_POINT('',(-79.8660249138713,105.235685467738,-74.8769043546876));
#3602=CARTESIAN_POINT('',(-71.8391803616632,98.7027402403375,-66.0708896394943));
#3603=CARTESIAN_POINT('Ctrl Pts',(-71.8391803616628,98.7027402403373,-66.070889639494));
#3604=CARTESIAN_POINT('Ctrl Pts',(-72.0439884445282,98.8361606209892,-66.3345813715533));
#3605=CARTESIAN_POINT('Ctrl Pts',(-72.2115336533623,99.001384056873,-66.6057676604154));
#3606=CARTESIAN_POINT('Ctrl Pts',(-72.5271374781293,99.4574342557344,-67.2436374185692));
#3607=CARTESIAN_POINT('Ctrl Pts',(-72.6502417628557,99.8096167014344,-67.645336798396));
#3608=CARTESIAN_POINT('Ctrl Pts',(-72.7143823519123,100.611874672149,-68.3522115825761));
#3609=CARTESIAN_POINT('Ctrl Pts',(-72.6558392149002,101.062790026477,-68.6563950132379));
#3610=CARTESIAN_POINT('Ctrl Pts',(-72.4034159189938,101.937209973525,-69.0936049867617));
#3611=CARTESIAN_POINT('Ctrl Pts',(-72.1935314433864,102.41615514562,-69.2543518193115));
#3612=CARTESIAN_POINT('Ctrl Pts',(-71.6369776563495,103.319666529344,-69.4003617123507));
#3613=CARTESIAN_POINT('Ctrl Pts',(-71.2897914679388,103.743726568121,-69.3867835747619));
#3614=CARTESIAN_POINT('Ctrl Pts',(-70.5589898894586,104.424395182907,-69.2374994608244));
#3615=CARTESIAN_POINT('Ctrl Pts',(-70.1256610955174,104.727134811084,-69.0917727209338));
#3616=CARTESIAN_POINT('Ctrl Pts',(-69.2156180135337,105.133251025888,-68.6985515492242));
#3617=CARTESIAN_POINT('Ctrl Pts',(-68.7380142610207,105.235685467739,-68.4521444087194));
#3618=CARTESIAN_POINT('Ctrl Pts',(-68.3007244674181,105.235685467739,-68.1996750286692));
#3619=CARTESIAN_POINT('Ctrl Pts',(-70.3007244674178,98.3074822374626,-64.7355734135318));
#3620=CARTESIAN_POINT('Ctrl Pts',(-70.7380142610204,98.3074822374626,-64.9880427935821));
#3621=CARTESIAN_POINT('Ctrl Pts',(-71.1649108408744,98.3807025943189,-65.3222773334404));
#3622=CARTESIAN_POINT('Ctrl Pts',(-71.63264360737,98.5810373096057,-65.817727530853));
#3623=CARTESIAN_POINT('Ctrl Pts',(-71.7401949633927,98.6382570943041,-65.9434452986592));
#3624=CARTESIAN_POINT('Ctrl Pts',(-71.8391803616628,98.7027402403373,-66.070889639494));
#3625=CARTESIAN_POINT('Origin',(-119.078493020361,109.,-80.7499999999988));
#3626=CARTESIAN_POINT('',(-93.4118265169985,98.3074822374623,-78.0787744031255));
#3627=CARTESIAN_POINT('',(-93.4118265169985,98.3074822374623,-78.0787744031255));
#3628=CARTESIAN_POINT('',(-89.310545785853,100.004330985067,-77.4236234448516));
#3629=CARTESIAN_POINT('Ctrl Pts',(-89.3105457858516,100.004330985068,-77.4236234448524));
#3630=CARTESIAN_POINT('Ctrl Pts',(-89.5906127684196,99.7001003271067,-77.3220467399197));
#3631=CARTESIAN_POINT('Ctrl Pts',(-89.9201573466291,99.432691593161,-77.2594832131444));
#3632=CARTESIAN_POINT('Ctrl Pts',(-90.7270152190322,98.9178350153006,-77.2137926604239));
#3633=CARTESIAN_POINT('Ctrl Pts',(-91.275429932033,98.6785063270153,-77.2683334201939));
#3634=CARTESIAN_POINT('Ctrl Pts',(-92.3773154492341,98.3741443355135,-77.5617079439358));
#3635=CARTESIAN_POINT('Ctrl Pts',(-92.930279409063,98.3074822374625,-77.8007530507317));
#3636=CARTESIAN_POINT('Ctrl Pts',(-93.4118265169985,98.3074822374625,-78.0787744031257));
#3637=CARTESIAN_POINT('',(-91.4118265169984,105.235685467738,-81.5428760182629));
#3638=CARTESIAN_POINT('Ctrl Pts',(-91.4118265169984,105.235685467738,-81.5428760182628));
#3639=CARTESIAN_POINT('Ctrl Pts',(-90.930279409063,105.235685467738,-81.2648546658689));
#3640=CARTESIAN_POINT('Ctrl Pts',(-90.4235466956197,105.142197830515,-80.9457346914359));
#3641=CARTESIAN_POINT('Ctrl Pts',(-89.5276720287663,104.732917302591,-80.2955389079813));
#3642=CARTESIAN_POINT('Ctrl Pts',(-89.1396330959697,104.416687991642,-79.9632191485941));
#3643=CARTESIAN_POINT('Ctrl Pts',(-88.6191933845126,103.711566927935,-79.3777677293152));
#3644=CARTESIAN_POINT('Ctrl Pts',(-88.4360002798934,103.294551166156,-79.0871156461153));
#3645=CARTESIAN_POINT('Ctrl Pts',(-88.2882811646739,102.403958803926,-78.5394916564604));
#3646=CARTESIAN_POINT('Ctrl Pts',(-88.3237355082,101.931198710495,-78.281198278488));
#3647=CARTESIAN_POINT('Ctrl Pts',(-88.5726881997782,101.068801289506,-77.8499995679938));
#3648=CARTESIAN_POINT('Ctrl Pts',(-88.8022989313345,100.623349028228,-77.6491867686112));
#3649=CARTESIAN_POINT('Ctrl Pts',(-89.1799219644913,100.151183250598,-77.4741046930827));
#3650=CARTESIAN_POINT('Ctrl Pts',(-89.2438824969059,100.076745862652,-77.4478013653234));
#3651=CARTESIAN_POINT('Ctrl Pts',(-89.3105457858516,100.004330985068,-77.4236234448524));
#3652=CARTESIAN_POINT('',(-91.4118265169984,105.235685467738,-81.5428760182629));
#3653=CARTESIAN_POINT('Ctrl Pts',(-81.8660249138711,98.3074822374626,-71.4128027395504));
#3654=CARTESIAN_POINT('Ctrl Pts',(-82.3237270253547,98.3074822374626,-71.6770571768241));
#3655=CARTESIAN_POINT('Ctrl Pts',(-82.7726916110599,98.3818254132719,-72.0253258196487));
#3656=CARTESIAN_POINT('Ctrl Pts',(-83.5294587228727,98.6836749369366,-72.8018086256385));
#3657=CARTESIAN_POINT('Ctrl Pts',(-83.8381825657519,98.9117809702808,-73.2288909422442));
#3658=CARTESIAN_POINT('Ctrl Pts',(-84.2642108337661,99.4513482675956,-74.0139591549906));
#3659=CARTESIAN_POINT('Ctrl Pts',(-84.4147303979509,99.7982897132532,-74.427397105883));
#3660=CARTESIAN_POINT('Ctrl Pts',(-84.5187012892031,100.598975519632,-75.1573598769691));
#3661=CARTESIAN_POINT('Ctrl Pts',(-84.4719272936971,101.053974393027,-75.4725395573331));
#3662=CARTESIAN_POINT('Ctrl Pts',(-84.2144142894456,101.946025606974,-75.9185651643065));
#3663=CARTESIAN_POINT('Ctrl Pts',(-83.9900828414982,102.430163538118,-76.072953886212));
#3664=CARTESIAN_POINT('Ctrl Pts',(-83.3943596113716,103.332957803082,-76.1947311507971));
#3665=CARTESIAN_POINT('Ctrl Pts',(-83.022912997837,103.751330105905,-76.1639500741449));
#3666=CARTESIAN_POINT('Ctrl Pts',(-82.2465265160762,104.425439262707,-75.9857200884568));
#3667=CARTESIAN_POINT('Ctrl Pts',(-81.7851543098186,104.72612267149,-75.8230324929145));
#3668=CARTESIAN_POINT('Ctrl Pts',(-80.8241649502783,105.131719766025,-75.4002729960248));
#3669=CARTESIAN_POINT('Ctrl Pts',(-80.3237270253549,105.235685467738,-75.1411587919613));
#3670=CARTESIAN_POINT('Ctrl Pts',(-79.8660249138712,105.235685467738,-74.8769043546876));
#3671=CARTESIAN_POINT('Origin',(-119.078493020361,109.,-80.7499999999988));
#3672=CARTESIAN_POINT('',(-104.90435628947,98.3074822374622,-84.7139895609318));
#3673=CARTESIAN_POINT('',(-104.90435628947,98.3074822374623,-84.7139895609318));
#3674=CARTESIAN_POINT('',(-99.9488699419194,100.228885141061,-83.7562504402684));
#3675=CARTESIAN_POINT('Ctrl Pts',(-99.9488699419193,100.228885141061,-83.7562504402685));
#3676=CARTESIAN_POINT('Ctrl Pts',(-100.269274778488,99.8589135037763,-83.6332987009061));
#3677=CARTESIAN_POINT('Ctrl Pts',(-100.672060551272,99.5388009858237,-83.5687616798079));
#3678=CARTESIAN_POINT('Ctrl Pts',(-101.656557156406,98.9446450743508,-83.5546921849167));
#3679=CARTESIAN_POINT('Ctrl Pts',(-102.323796076877,98.6892023001508,-83.659021954752));
#3680=CARTESIAN_POINT('Ctrl Pts',(-103.656688844209,98.3714816818226,-84.070990296531));
#3681=CARTESIAN_POINT('Ctrl Pts',(-104.322168303632,98.3074822374624,-84.3778631705889));
#3682=CARTESIAN_POINT('Ctrl Pts',(-104.90435628947,98.3074822374624,-84.7139895609318));
#3683=CARTESIAN_POINT('',(-102.90435628947,105.235685467738,-88.1780911760691));
#3684=CARTESIAN_POINT('Ctrl Pts',(-102.90435628947,105.235685467738,-88.178091176069));
#3685=CARTESIAN_POINT('Ctrl Pts',(-102.322168303632,105.235685467738,-87.8419647857261));
#3686=CARTESIAN_POINT('Ctrl Pts',(-101.701146422792,105.145679342323,-87.4580891267805));
#3687=CARTESIAN_POINT('Ctrl Pts',(-100.583248552382,104.718635790978,-86.6737387001651));
#3688=CARTESIAN_POINT('Ctrl Pts',(-100.087436405043,104.380238803494,-86.2724890494876));
#3689=CARTESIAN_POINT('Ctrl Pts',(-99.4797157079115,103.63823946452,-85.6153691751923));
#3690=CARTESIAN_POINT('Ctrl Pts',(-99.2762414496599,103.243002384244,-85.320427254354));
#3691=CARTESIAN_POINT('Ctrl Pts',(-99.0952115751188,102.385815407921,-84.7678773474479));
#3692=CARTESIAN_POINT('Ctrl Pts',(-99.1179825761209,101.924673720388,-84.5089097354468));
#3693=CARTESIAN_POINT('Ctrl Pts',(-99.3631680629044,101.075326279613,-84.0842360150593));
#3694=CARTESIAN_POINT('Ctrl Pts',(-99.5989917777891,100.640669594177,-83.8953044405758));
#3695=CARTESIAN_POINT('Ctrl Pts',(-99.9319639746297,100.248502859387,-83.7627974003584));
#3696=CARTESIAN_POINT('Ctrl Pts',(-99.940389585881,100.238677412744,-83.7595046811735));
#3697=CARTESIAN_POINT('Ctrl Pts',(-99.9488699419193,100.228885141061,-83.7562504402685));
#3698=CARTESIAN_POINT('',(-102.90435628947,105.235685467738,-88.1780911760691));
#3699=CARTESIAN_POINT('Ctrl Pts',(-93.4118265169985,98.3074822374625,-78.0787744031257));
#3700=CARTESIAN_POINT('Ctrl Pts',(-93.9211136281798,98.3074822374625,-78.372811453861));
#3701=CARTESIAN_POINT('Ctrl Pts',(-94.4293110479316,98.3809411378057,-78.7542137874603));
#3702=CARTESIAN_POINT('Ctrl Pts',(-95.3131003585774,98.6801492903014,-79.6011997737382));
#3703=CARTESIAN_POINT('Ctrl Pts',(-95.68953602647,98.9062732240902,-80.0657700699796));
#3704=CARTESIAN_POINT('Ctrl Pts',(-96.2180755930993,99.439773757549,-80.9039616912801));
#3705=CARTESIAN_POINT('Ctrl Pts',(-96.4211158671793,99.7760817327783,-81.3392544545395));
#3706=CARTESIAN_POINT('Ctrl Pts',(-96.603988459357,100.572512615503,-82.1140272198499));
#3707=CARTESIAN_POINT('Ctrl Pts',(-96.5825452086925,101.034655609006,-82.4517288812605));
#3708=CARTESIAN_POINT('Ctrl Pts',(-96.3138784992858,101.965344390996,-82.9170732722552));
#3709=CARTESIAN_POINT('Ctrl Pts',(-96.0594130029196,102.458977333713,-83.0572595789545));
#3710=CARTESIAN_POINT('Ctrl Pts',(-95.3867915721352,103.359086193817,-83.1307566850585));
#3711=CARTESIAN_POINT('Ctrl Pts',(-94.9692620595266,103.765790736204,-83.0669701806072));
#3712=CARTESIAN_POINT('Ctrl Pts',(-94.0943036219507,104.432320373106,-82.8287936444868));
#3713=CARTESIAN_POINT('Ctrl Pts',(-93.5664254574151,104.730808636538,-82.6265294468561));
#3714=CARTESIAN_POINT('Ctrl Pts',(-92.4801710348681,105.132960205189,-82.130223321151));
#3715=CARTESIAN_POINT('Ctrl Pts',(-91.9211136281798,105.235685467738,-81.8369130689982));
#3716=CARTESIAN_POINT('Ctrl Pts',(-91.4118265169984,105.235685467738,-81.5428760182629));
#3717=CARTESIAN_POINT('Origin',(-119.078493020361,109.,-80.7499999999988));
#3718=CARTESIAN_POINT('',(-106.270002469182,105.235685467738,-90.1212479039226));
#3719=CARTESIAN_POINT('',(-106.270002469182,105.235685467738,-90.1212479039226));
#3720=CARTESIAN_POINT('Ctrl Pts',(-104.90435628947,98.3074822374624,-84.7139895609318));
#3721=CARTESIAN_POINT('Ctrl Pts',(-105.520546937821,98.3074822374624,-85.0697473976293));
#3722=CARTESIAN_POINT('Ctrl Pts',(-106.150726410955,98.3786464989181,-85.5188532090103));
#3723=CARTESIAN_POINT('Ctrl Pts',(-107.289220969567,98.6734920739597,-86.5082604731963));
#3724=CARTESIAN_POINT('Ctrl Pts',(-107.798461931632,98.8969623992174,-87.0475589280851));
#3725=CARTESIAN_POINT('Ctrl Pts',(-108.520316145588,99.4223913020677,-87.9892961628252));
#3726=CARTESIAN_POINT('Ctrl Pts',(-108.815648667087,99.7399146036544,-88.4622960553437));
#3727=CARTESIAN_POINT('Ctrl Pts',(-109.06520359177,100.328003547478,-89.1041494241911));
#3728=CARTESIAN_POINT('Ctrl Pts',(-109.116864532686,100.542611823444,-89.3070609778502));
#3729=CARTESIAN_POINT('Ctrl Pts',(-109.140178467765,101.001678002652,-89.6682684715672));
#3730=CARTESIAN_POINT('Ctrl Pts',(-109.111806983136,101.246175947599,-89.8265150985448));
#3731=CARTESIAN_POINT('Ctrl Pts',(-108.965261598155,101.753824052402,-90.080339150946));
#3732=CARTESIAN_POINT('Ctrl Pts',(-108.849954531701,102.007043208325,-90.1709510744033));
#3733=CARTESIAN_POINT('Ctrl Pts',(-108.552569635501,102.497386688197,-90.2844484102263));
#3734=CARTESIAN_POINT('Ctrl Pts',(-108.370506562727,102.734504647816,-90.3073999743598));
#3735=CARTESIAN_POINT('Ctrl Pts',(-107.75853069038,103.401878694155,-90.2932781005938));
#3736=CARTESIAN_POINT('Ctrl Pts',(-107.260215630608,103.787507531247,-90.1718542774143));
#3737=CARTESIAN_POINT('Ctrl Pts',(-106.197183712277,104.44395286517,-89.8210541610607));
#3738=CARTESIAN_POINT('Ctrl Pts',(-105.538070840598,104.739654064067,-89.5413414682492));
#3739=CARTESIAN_POINT('Ctrl Pts',(-104.200003266355,105.136149694813,-88.8976048069571));
#3740=CARTESIAN_POINT('Ctrl Pts',(-103.520546937821,105.235685467738,-88.5338490127664));
#3741=CARTESIAN_POINT('Ctrl Pts',(-102.90435628947,105.235685467738,-88.178091176069));
#3742=CARTESIAN_POINT('',(-108.270002469182,98.3074822374624,-86.6571462887851));
#3743=CARTESIAN_POINT('',(-108.270002469182,98.3074822374623,-86.6571462887851));
#3744=CARTESIAN_POINT('Ctrl Pts',(-106.270002469182,105.235685467738,-90.1212479039226));
#3745=CARTESIAN_POINT('Ctrl Pts',(-106.398364251285,105.235685467738,-90.1953576133737));
#3746=CARTESIAN_POINT('Ctrl Pts',(-106.527960736738,105.218918283964,-90.2651932010029));
#3747=CARTESIAN_POINT('Ctrl Pts',(-106.847366026658,105.139174343852,-90.425397613589));
#3748=CARTESIAN_POINT('Ctrl Pts',(-107.033287150629,105.059113530962,-90.5082215504996));
#3749=CARTESIAN_POINT('Ctrl Pts',(-107.487244640969,104.791037335221,-90.6836023495469));
#3750=CARTESIAN_POINT('Ctrl Pts',(-107.742055343965,104.569575136487,-90.7553778221103));
#3751=CARTESIAN_POINT('Ctrl Pts',(-108.312044999287,103.952474510198,-90.8506321914898));
#3752=CARTESIAN_POINT('Ctrl Pts',(-108.601687275107,103.516179693072,-90.83222067748));
#3753=CARTESIAN_POINT('Ctrl Pts',(-109.016285784176,102.748005272445,-90.6902990309755));
#3754=CARTESIAN_POINT('Ctrl Pts',(-109.166799177582,102.411600006565,-90.5937735724328));
#3755=CARTESIAN_POINT('Ctrl Pts',(-109.364309285276,101.886060973467,-90.3923049613581));
#3756=CARTESIAN_POINT('Ctrl Pts',(-109.428881856401,101.691891969437,-90.3067091143765));
#3757=CARTESIAN_POINT('Ctrl Pts',(-109.539343060738,101.309363471567,-90.1154913997023));
#3758=CARTESIAN_POINT('Ctrl Pts',(-109.58547134865,101.12019828098,-90.0094768684831));
#3759=CARTESIAN_POINT('Ctrl Pts',(-109.683806016576,100.621556930253,-89.6991065970049));
#3760=CARTESIAN_POINT('Ctrl Pts',(-109.718746169311,100.316400657043,-89.4751827475122));
#3761=CARTESIAN_POINT('Ctrl Pts',(-109.719931149862,99.6457292128168,-88.8981274115455));
#3762=CARTESIAN_POINT('Ctrl Pts',(-109.659507933391,99.2872907854466,-88.5188240602725));
#3763=CARTESIAN_POINT('Ctrl Pts',(-109.407078555524,98.8025861049536,-87.8721136642323));
#3764=CARTESIAN_POINT('Ctrl Pts',(-109.264504916411,98.6353091816041,-87.6059682053067));
#3765=CARTESIAN_POINT('Ctrl Pts',(-108.94540320403,98.4361359224893,-87.1969059803222));
#3766=CARTESIAN_POINT('Ctrl Pts',(-108.799409958408,98.3776732407719,-87.0447641078801));
#3767=CARTESIAN_POINT('Ctrl Pts',(-108.519683286228,98.3196123402596,-86.8155806823361));
#3768=CARTESIAN_POINT('Ctrl Pts',(-108.39839753492,98.3074822374624,-86.7312752145517));
#3769=CARTESIAN_POINT('Ctrl Pts',(-108.270002469182,98.3074822374624,-86.6571462887851));
#3770=CARTESIAN_POINT('Origin',(-119.078493020361,109.,-80.7499999999988));
#3771=CARTESIAN_POINT('',(-85.1260169266464,123.456832294801,-65.7663309411545));
#3772=CARTESIAN_POINT('',(-73.5607164801933,123.456832294801,-59.0891016151359));
#3773=CARTESIAN_POINT('',(-85.1260169266463,123.456832294801,-65.7663309411548));
#3774=CARTESIAN_POINT('',(-83.1162922298706,123.872941359692,-62.2368404208554));
#3775=CARTESIAN_POINT('Ctrl Pts',(-83.1162922298706,123.872941359692,-62.2368404208554));
#3776=CARTESIAN_POINT('Ctrl Pts',(-83.1062743831766,123.829770440363,-62.6116107413721));
#3777=CARTESIAN_POINT('Ctrl Pts',(-83.1509026868771,123.7792071983,-62.9828538443025));
#3778=CARTESIAN_POINT('Ctrl Pts',(-83.3664532434541,123.66173721786,-63.8135927138417));
#3779=CARTESIAN_POINT('Ctrl Pts',(-83.6030554954123,123.587986446344,-64.3071289633042));
#3780=CARTESIAN_POINT('Ctrl Pts',(-84.2623538476765,123.484750532966,-65.1560397594667));
#3781=CARTESIAN_POINT('Ctrl Pts',(-84.6849506657898,123.456832294801,-65.5116812167184));
#3782=CARTESIAN_POINT('Ctrl Pts',(-85.1260169266465,123.456832294801,-65.7663309411545));
#3783=CARTESIAN_POINT('',(-89.1260169266464,123.456832294801,-58.8381277108788));
#3784=CARTESIAN_POINT('Ctrl Pts',(-89.1260169266463,123.456832294801,-58.8381277108789));
#3785=CARTESIAN_POINT('Ctrl Pts',(-88.6849506657896,123.456832294801,-58.5834779864428));
#3786=CARTESIAN_POINT('Ctrl Pts',(-88.165657720114,123.484750532965,-58.395319135024));
#3787=CARTESIAN_POINT('Ctrl Pts',(-87.1008302289584,123.587986446343,-58.2488054113713));
#3788=CARTESIAN_POINT('Ctrl Pts',(-86.5551141732562,123.66173721786,-58.2906699753141));
#3789=CARTESIAN_POINT('Ctrl Pts',(-85.5888213740156,123.798956955934,-58.5578170932871));
#3790=CARTESIAN_POINT('Ctrl Pts',(-85.1044718647574,123.871021105468,-58.7975024013151));
#3791=CARTESIAN_POINT('Ctrl Pts',(-84.2687404142013,123.972199967385,-59.4532843052146));
#3792=CARTESIAN_POINT('Ctrl Pts',(-83.9170521365101,124.,-59.8691926348772));
#3793=CARTESIAN_POINT('Ctrl Pts',(-83.4144629487118,124.,-60.7397026434787));
#3794=CARTESIAN_POINT('Ctrl Pts',(-83.2301199084241,123.972199967385,-61.2522277910038));
#3795=CARTESIAN_POINT('Ctrl Pts',(-83.1333491468145,123.906950854201,-61.9304287037879));
#3796=CARTESIAN_POINT('Ctrl Pts',(-83.120379607442,123.890555509,-62.0839305341979));
#3797=CARTESIAN_POINT('Ctrl Pts',(-83.1162922298706,123.872941359692,-62.2368404208553));
#3798=CARTESIAN_POINT('',(-77.5607164801934,123.456832294801,-52.1608983848601));
#3799=CARTESIAN_POINT('',(-89.1260169266463,123.456832294801,-58.8381277108789));
#3800=CARTESIAN_POINT('',(-75.5607164801928,123.594519519327,-59.6249999999981));
#3801=CARTESIAN_POINT('Ctrl Pts',(-75.5607164801923,123.594519519327,-59.6249999999981));
#3802=CARTESIAN_POINT('Ctrl Pts',(-75.9177670555452,123.636893626714,-59.6249999999981));
#3803=CARTESIAN_POINT('Ctrl Pts',(-76.270167318939,123.685122421852,-59.576007942327));
#3804=CARTESIAN_POINT('Ctrl Pts',(-77.0792037993761,123.798839176147,-59.3592272707466));
#3805=CARTESIAN_POINT('Ctrl Pts',(-77.5695548504124,123.870716769224,-59.1248365924091));
#3806=CARTESIAN_POINT('Ctrl Pts',(-78.4161592503826,123.971970182233,-58.476444301003));
#3807=CARTESIAN_POINT('Ctrl Pts',(-78.7723947994248,124.,-58.0622099735219));
#3808=CARTESIAN_POINT('Ctrl Pts',(-79.2772413912376,124.,-57.1877900264742));
#3809=CARTESIAN_POINT('Ctrl Pts',(-79.4578610674346,123.971970182233,-56.672163827532));
#3810=CARTESIAN_POINT('Ctrl Pts',(-79.5960830634252,123.870716769223,-55.6147867644991));
#3811=CARTESIAN_POINT('Ctrl Pts',(-79.5538958197575,123.798839176147,-55.0729349583605));
#3812=CARTESIAN_POINT('Ctrl Pts',(-79.2949201129009,123.662988149345,-54.1064244624455));
#3813=CARTESIAN_POINT('Ctrl Pts',(-79.0605274269875,123.589960152211,-53.6161302759907));
#3814=CARTESIAN_POINT('Ctrl Pts',(-78.4121993371972,123.486046379795,-52.7696054406997));
#3815=CARTESIAN_POINT('Ctrl Pts',(-77.9980062737959,123.456832294801,-52.4133677649104));
#3816=CARTESIAN_POINT('Ctrl Pts',(-77.5607164801933,123.456832294801,-52.1608983848601));
#3817=CARTESIAN_POINT('Ctrl Pts',(-73.5607164801933,123.456832294801,-59.0891016151359));
#3818=CARTESIAN_POINT('Ctrl Pts',(-73.9980062737958,123.456832294801,-59.3415709951862));
#3819=CARTESIAN_POINT('Ctrl Pts',(-74.5136136825151,123.486046379796,-59.5221538722684));
#3820=CARTESIAN_POINT('Ctrl Pts',(-75.214498480876,123.554932441228,-59.6137729046024));
#3821=CARTESIAN_POINT('Ctrl Pts',(-75.3881510574346,123.57403977147,-59.6249999999981));
#3822=CARTESIAN_POINT('Ctrl Pts',(-75.5607164801923,123.594519519327,-59.6249999999981));
#3823=CARTESIAN_POINT('Origin',(-119.078493020361,109.,-80.7499999999988));
#3824=CARTESIAN_POINT('',(-96.6718185297735,123.456832294801,-72.4323026047302));
#3825=CARTESIAN_POINT('',(-96.6718185297736,123.456832294801,-72.4323026047302));
#3826=CARTESIAN_POINT('',(-94.4177421038261,123.892951352905,-68.5776999378933));
#3827=CARTESIAN_POINT('Ctrl Pts',(-94.4177421038264,123.892951352906,-68.5776999378912));
#3828=CARTESIAN_POINT('Ctrl Pts',(-94.3950722235507,123.847611592354,-69.0004788607279));
#3829=CARTESIAN_POINT('Ctrl Pts',(-94.4446100038828,123.791696326041,-69.4229013343407));
#3830=CARTESIAN_POINT('Ctrl Pts',(-94.6962798517419,123.665476993059,-70.3388246478844));
#3831=CARTESIAN_POINT('Ctrl Pts',(-94.9708319480395,123.588576370395,-70.867709374078));
#3832=CARTESIAN_POINT('Ctrl Pts',(-95.7182701307845,123.483657833973,-71.7750046897054));
#3833=CARTESIAN_POINT('Ctrl Pts',(-96.1902714218383,123.456832294801,-72.154281252336));
#3834=CARTESIAN_POINT('Ctrl Pts',(-96.6718185297737,123.456832294801,-72.43230260473));
#3835=CARTESIAN_POINT('',(-100.671818529773,123.456832294801,-65.5040993744542));
#3836=CARTESIAN_POINT('Ctrl Pts',(-100.671818529773,123.456832294801,-65.5040993744543));
#3837=CARTESIAN_POINT('Ctrl Pts',(-100.198890562852,123.456832294801,-65.2310542854448));
#3838=CARTESIAN_POINT('Ctrl Pts',(-99.6449352638787,123.482663841571,-65.0141879033647));
#3839=CARTESIAN_POINT('Ctrl Pts',(-98.5058533293481,123.584301615867,-64.8160574918001));
#3840=CARTESIAN_POINT('Ctrl Pts',(-97.9204236427471,123.659016564532,-64.8359793331119));
#3841=CARTESIAN_POINT('Ctrl Pts',(-96.9056954794152,123.797787553474,-65.0846768377439));
#3842=CARTESIAN_POINT('Ctrl Pts',(-96.4098673945079,123.869713255231,-65.3135356756117));
#3843=CARTESIAN_POINT('Ctrl Pts',(-95.5559638106463,123.971567821815,-65.9593477666097));
#3844=CARTESIAN_POINT('Ctrl Pts',(-95.1973252908835,124.,-66.3757915444938));
#3845=CARTESIAN_POINT('Ctrl Pts',(-94.6944496907949,124.,-67.2467976337339));
#3846=CARTESIAN_POINT('Ctrl Pts',(-94.5146381715445,123.972692167848,-67.755124974498));
#3847=CARTESIAN_POINT('Ctrl Pts',(-94.4324796442889,123.913947930132,-68.376407921987));
#3848=CARTESIAN_POINT('Ctrl Pts',(-94.4231381300388,123.903743405331,-68.4770674633497));
#3849=CARTESIAN_POINT('Ctrl Pts',(-94.4177421038264,123.892951352906,-68.5776999378912));
#3850=CARTESIAN_POINT('',(-100.671818529773,123.456832294801,-65.5040993744543));
#3851=CARTESIAN_POINT('Ctrl Pts',(-85.1260169266465,123.456832294801,-65.7663309411545));
#3852=CARTESIAN_POINT('Ctrl Pts',(-85.5837190381301,123.456832294801,-66.0305853784282));
#3853=CARTESIAN_POINT('Ctrl Pts',(-86.122720562641,123.486454820705,-66.2229054686833));
#3854=CARTESIAN_POINT('Ctrl Pts',(-87.2307450620227,123.590202391576,-66.3909926328699));
#3855=CARTESIAN_POINT('Ctrl Pts',(-87.7998683754043,123.662779767014,-66.3670498363015));
#3856=CARTESIAN_POINT('Ctrl Pts',(-88.8096922981326,123.797321626501,-66.140954313845));
#3857=CARTESIAN_POINT('Ctrl Pts',(-89.3225329048017,123.868752483667,-65.9268338105032));
#3858=CARTESIAN_POINT('Ctrl Pts',(-90.208346563904,123.970860942253,-65.3026051841426));
#3859=CARTESIAN_POINT('Ctrl Pts',(-90.5808483157038,124.,-64.8915779677916));
#3860=CARTESIAN_POINT('Ctrl Pts',(-91.095874324207,124.,-63.9995267538447));
#3861=CARTESIAN_POINT('Ctrl Pts',(-91.2655834593138,123.970860942253,-63.4714171656563));
#3862=CARTESIAN_POINT('Ctrl Pts',(-91.3632744779603,123.868752483666,-62.3921657206742));
#3863=CARTESIAN_POINT('Ctrl Pts',(-91.2922879699909,123.797321626501,-61.8409724755356));
#3864=CARTESIAN_POINT('Ctrl Pts',(-90.9831804747559,123.662779767014,-60.8533915438754));
#3865=CARTESIAN_POINT('Ctrl Pts',(-90.7193538881309,123.590202391575,-60.3485448983168));
#3866=CARTESIAN_POINT('Ctrl Pts',(-90.0197738842044,123.486454820704,-59.47301111593));
#3867=CARTESIAN_POINT('Ctrl Pts',(-89.5837190381299,123.456832294801,-59.1023821481526));
#3868=CARTESIAN_POINT('Ctrl Pts',(-89.1260169266463,123.456832294801,-58.8381277108788));
#3869=CARTESIAN_POINT('Origin',(-119.078493020361,109.,-80.7499999999988));
#3870=CARTESIAN_POINT('',(-108.164348302245,123.456832294801,-79.0675177625366));
#3871=CARTESIAN_POINT('',(-108.164348302245,123.456832294801,-79.0675177625365));
#3872=CARTESIAN_POINT('',(-105.277091391218,123.923615035047,-74.5275001761057));
#3873=CARTESIAN_POINT('Ctrl Pts',(-105.277091391218,123.923615035047,-74.5275001761056));
#3874=CARTESIAN_POINT('Ctrl Pts',(-105.275365738248,123.921622422635,-74.5492158639596));
#3875=CARTESIAN_POINT('Ctrl Pts',(-105.273837242761,123.919598892701,-74.5709499461767));
#3876=CARTESIAN_POINT('Ctrl Pts',(-105.238853605271,123.865658954398,-75.1423248070353));
#3877=CARTESIAN_POINT('Ctrl Pts',(-105.33860750079,123.794453706366,-75.701175262549));
#3878=CARTESIAN_POINT('Ctrl Pts',(-105.746737061739,123.654133883405,-76.7806745481755));
#3879=CARTESIAN_POINT('Ctrl Pts',(-106.120272716169,123.5787523934,-77.3509626000236));
#3880=CARTESIAN_POINT('Ctrl Pts',(-107.054281271328,123.479989785222,-78.3346823431572));
#3881=CARTESIAN_POINT('Ctrl Pts',(-107.613395871184,123.456832294801,-78.7494252281526));
#3882=CARTESIAN_POINT('Ctrl Pts',(-108.164348302246,123.456832294801,-79.0675177625365));
#3883=CARTESIAN_POINT('',(-112.164348302245,123.456832294801,-72.1393145322606));
#3884=CARTESIAN_POINT('Ctrl Pts',(-112.164348302245,123.456832294801,-72.1393145322606));
#3885=CARTESIAN_POINT('Ctrl Pts',(-111.613395871184,123.456832294801,-71.8212219978767));
#3886=CARTESIAN_POINT('Ctrl Pts',(-110.974660696811,123.479989785221,-71.5443859932717));
#3887=CARTESIAN_POINT('Ctrl Pts',(-109.655730131473,123.578752393399,-71.2273707287195));
#3888=CARTESIAN_POINT('Ctrl Pts',(-108.975078363883,123.654133883405,-71.1890233886878));
#3889=CARTESIAN_POINT('Ctrl Pts',(-107.836139778689,123.794453706366,-71.3753224636836));
#3890=CARTESIAN_POINT('Ctrl Pts',(-107.302284139538,123.865658954397,-71.5683582837951));
#3891=CARTESIAN_POINT('Ctrl Pts',(-106.383953947217,123.96943271423,-72.1762726463728));
#3892=CARTESIAN_POINT('Ctrl Pts',(-105.998960269092,124.,-72.5907067654734));
#3893=CARTESIAN_POINT('Ctrl Pts',(-105.482985495051,124.,-73.4844012895352));
#3894=CARTESIAN_POINT('Ctrl Pts',(-105.318978111356,123.971981653342,-74.0003959692113));
#3895=CARTESIAN_POINT('Ctrl Pts',(-105.277091391218,123.923615035047,-74.5275001761056));
#3896=CARTESIAN_POINT('',(-112.164348302245,123.456832294801,-72.1393145322605));
#3897=CARTESIAN_POINT('Ctrl Pts',(-96.6718185297737,123.456832294801,-72.43230260473));
#3898=CARTESIAN_POINT('Ctrl Pts',(-97.2080109095617,123.456832294801,-72.741873419538));
#3899=CARTESIAN_POINT('Ctrl Pts',(-97.8378331599511,123.489300624785,-72.9756291788421));
#3900=CARTESIAN_POINT('Ctrl Pts',(-99.1346770015159,123.601479985038,-73.210267194341));
#3901=CARTESIAN_POINT('Ctrl Pts',(-99.801733680399,123.679673134231,-73.2116784585455));
#3902=CARTESIAN_POINT('Ctrl Pts',(-100.899904621245,123.812998388381,-73.0077930813484));
#3903=CARTESIAN_POINT('Ctrl Pts',(-101.417162434113,123.877803175384,-72.8258148556167));
#3904=CARTESIAN_POINT('Ctrl Pts',(-102.313026843884,123.972069837582,-72.2590940486296));
#3905=CARTESIAN_POINT('Ctrl Pts',(-102.69054002654,124.,-71.8723715243807));
#3906=CARTESIAN_POINT('Ctrl Pts',(-103.196264738206,124.,-70.9964306291323));
#3907=CARTESIAN_POINT('Ctrl Pts',(-103.342419677093,123.972069837582,-70.4761333605637));
#3908=CARTESIAN_POINT('Ctrl Pts',(-103.385282087912,123.877803175384,-69.4169316198625));
#3909=CARTESIAN_POINT('Ctrl Pts',(-103.284250947897,123.812998388381,-68.8779841007473));
#3910=CARTESIAN_POINT('Ctrl Pts',(-102.911735393587,123.67967313423,-67.8249974796778));
#3911=CARTESIAN_POINT('Ctrl Pts',(-102.576984863492,123.601479985038,-67.2480150821033));
#3912=CARTESIAN_POINT('Ctrl Pts',(-101.725360460594,123.489300624784,-66.2422343783163));
#3913=CARTESIAN_POINT('Ctrl Pts',(-101.208010909561,123.456832294801,-65.8136701892623));
#3914=CARTESIAN_POINT('Ctrl Pts',(-100.671818529773,123.456832294801,-65.5040993744543));
#3915=CARTESIAN_POINT('Origin',(-119.078493020361,109.,-80.7499999999988));
#3916=CARTESIAN_POINT('',(-115.529994481957,123.456832294801,-74.0824712601142));
#3917=CARTESIAN_POINT('',(-115.529994481957,123.456832294801,-74.082471260114));
#3918=CARTESIAN_POINT('Ctrl Pts',(-108.164348302246,123.456832294801,-79.0675177625365));
#3919=CARTESIAN_POINT('Ctrl Pts',(-108.844463055017,123.456832294801,-79.4601821981288));
#3920=CARTESIAN_POINT('Ctrl Pts',(-109.637912977074,123.491441900927,-79.7804741154724));
#3921=CARTESIAN_POINT('Ctrl Pts',(-111.275183810088,123.611693066724,-80.170706138189));
#3922=CARTESIAN_POINT('Ctrl Pts',(-112.118571906507,123.696010228407,-80.2428658921871));
#3923=CARTESIAN_POINT('Ctrl Pts',(-113.398550856209,123.828649318389,-80.1045968599479));
#3924=CARTESIAN_POINT('Ctrl Pts',(-113.937605814753,123.885984825864,-79.974373351834));
#3925=CARTESIAN_POINT('Ctrl Pts',(-114.643393821985,123.950735654834,-79.6153146748024));
#3926=CARTESIAN_POINT('Ctrl Pts',(-114.862132214305,123.968740024147,-79.4686771786292));
#3927=CARTESIAN_POINT('Ctrl Pts',(-115.243722739859,123.993392806363,-79.1229603686417));
#3928=CARTESIAN_POINT('Ctrl Pts',(-115.406496999395,124.,-78.9237921724865));
#3929=CARTESIAN_POINT('Ctrl Pts',(-115.660952638663,124.,-78.4830620770019));
#3930=CARTESIAN_POINT('Ctrl Pts',(-115.752050226392,123.993392806363,-78.2425113350836));
#3931=CARTESIAN_POINT('Ctrl Pts',(-115.860654503579,123.968740024147,-77.7391858411162));
#3932=CARTESIAN_POINT('Ctrl Pts',(-115.878277104252,123.950735654834,-77.4764340884979));
#3933=CARTESIAN_POINT('Ctrl Pts',(-115.836337036395,123.885984825864,-76.6856744060329));
#3934=CARTESIAN_POINT('Ctrl Pts',(-115.679586423319,123.828649318388,-76.1537273638406));
#3935=CARTESIAN_POINT('Ctrl Pts',(-115.159341442944,123.696010228406,-74.9760985609694));
#3936=CARTESIAN_POINT('Ctrl Pts',(-114.675155214641,123.611693066724,-74.2817829212208));
#3937=CARTESIAN_POINT('Ctrl Pts',(-113.518568953091,123.491441900926,-73.0589807983134));
#3938=CARTESIAN_POINT('Ctrl Pts',(-112.844463055016,123.456832294801,-72.531978967853));
#3939=CARTESIAN_POINT('Ctrl Pts',(-112.164348302245,123.456832294801,-72.1393145322606));
#3940=CARTESIAN_POINT('',(-111.529994481957,123.456832294801,-81.0106744903897));
#3941=CARTESIAN_POINT('',(-111.529994481957,123.456832294801,-81.0106744903897));
#3942=CARTESIAN_POINT('Ctrl Pts',(-115.529994481957,123.456832294801,-74.0824712601142));
#3943=CARTESIAN_POINT('Ctrl Pts',(-115.65835626406,123.456832294801,-74.1565809695654));
#3944=CARTESIAN_POINT('Ctrl Pts',(-115.77745320865,123.461475653088,-74.2446022954246));
#3945=CARTESIAN_POINT('Ctrl Pts',(-116.046607194207,123.483194384997,-74.4918445203156));
#3946=CARTESIAN_POINT('Ctrl Pts',(-116.181936272838,123.504836535895,-74.6622964502142));
#3947=CARTESIAN_POINT('Ctrl Pts',(-116.463492476953,123.573840873615,-75.1362850362945));
#3948=CARTESIAN_POINT('Ctrl Pts',(-116.573472758241,123.62806730643,-75.4589141577373));
#3949=CARTESIAN_POINT('Ctrl Pts',(-116.724373411066,123.761245635907,-76.2800519723337));
#3950=CARTESIAN_POINT('Ctrl Pts',(-116.704520006728,123.840165624527,-76.7977027010819));
#3951=CARTESIAN_POINT('Ctrl Pts',(-116.53883398008,123.93828517935,-77.6608633532843));
#3952=CARTESIAN_POINT('Ctrl Pts',(-116.424541973442,123.968919507233,-78.0229943017362));
#3953=CARTESIAN_POINT('Ctrl Pts',(-116.189563012637,123.995063180093,-78.5706187310189));
#3954=CARTESIAN_POINT('Ctrl Pts',(-116.090247091074,123.99999005338,-78.7688860801498));
#3955=CARTESIAN_POINT('Ctrl Pts',(-115.86944609645,124.000009911765,-79.1514313247033));
#3956=CARTESIAN_POINT('Ctrl Pts',(-115.74750688821,123.995107474062,-79.3365182359193));
#3957=CARTESIAN_POINT('Ctrl Pts',(-115.391456612351,123.969070285569,-79.8131657732718));
#3958=CARTESIAN_POINT('Ctrl Pts',(-115.135714858818,123.938576005114,-80.0927177542768));
#3959=CARTESIAN_POINT('Ctrl Pts',(-114.471237782264,123.840607113622,-80.6686229218872));
#3960=CARTESIAN_POINT('Ctrl Pts',(-114.031900126614,123.761512834073,-80.9456186309926));
#3961=CARTESIAN_POINT('Ctrl Pts',(-113.24419775823,123.628137504237,-81.2260282504464));
#3962=CARTESIAN_POINT('Ctrl Pts',(-112.909789654842,123.573903068408,-81.292149830288));
#3963=CARTESIAN_POINT('Ctrl Pts',(-112.358412824606,123.504868123884,-81.2853999107625));
#3964=CARTESIAN_POINT('Ctrl Pts',(-112.143032917437,123.483209990156,-81.2534392614886));
#3965=CARTESIAN_POINT('Ctrl Pts',(-111.794203638433,123.461478073366,-81.1439450618975));
#3966=CARTESIAN_POINT('Ctrl Pts',(-111.658389547695,123.456832294801,-81.0848034161563));
#3967=CARTESIAN_POINT('Ctrl Pts',(-111.529994481957,123.456832294801,-81.0106744903897));
#3968=CARTESIAN_POINT('Origin',(-119.078493020361,109.,-80.7499999999988));
#3969=CARTESIAN_POINT('',(-126.564449609913,108.0824948189,-67.7839428436388));
#3970=CARTESIAN_POINT('',(-122.424179917669,122.42480974691,-74.9551003076436));
#3971=CARTESIAN_POINT('Origin',(-119.078493020361,109.,-80.7499999999988));
#3972=CARTESIAN_POINT('',(-77.2010015942,108.0824948189,-39.2839428436393));
#3973=CARTESIAN_POINT('',(-126.564449609913,108.0824948189,-67.7839428436388));
#3974=CARTESIAN_POINT('',(-73.0607319019557,122.42480974691,-46.4551003076441));
#3975=CARTESIAN_POINT('Origin',(-69.7150450046476,109.,-52.2499999999992));
#3976=CARTESIAN_POINT('',(-122.424179917669,122.42480974691,-74.9551003076436));
#3977=CARTESIAN_POINT('Origin',(-69.7150450046476,109.,-52.2499999999992));
#3978=CARTESIAN_POINT('',(-73.7335498795933,101.937180526609,-39.2897453861299));
#3979=CARTESIAN_POINT('',(-70.2694482644555,101.937180526609,-37.2897453861299));
#3980=CARTESIAN_POINT('',(-73.7335498795933,101.937180526609,-39.2897453861299));
#3981=CARTESIAN_POINT('',(-67.366968793295,123.991664350565,-50.3169872981059));
#3982=CARTESIAN_POINT('Origin',(-67.1169687932943,109.,-50.7499999999993));
#3983=CARTESIAN_POINT('',(-63.9028671781572,123.991664350565,-48.3169872981059));
#3984=CARTESIAN_POINT('',(-67.366968793295,123.991664350565,-50.3169872981059));
#3985=CARTESIAN_POINT('Origin',(-63.6528671781565,109.,-48.7499999999993));
#3986=CARTESIAN_POINT('Origin',(-69.7150450046476,109.,-52.2499999999992));
#3987=CARTESIAN_POINT('',(-78.2150450046475,109.,-37.5275681356637));
#3988=CARTESIAN_POINT('Origin',(-69.7150450046476,109.,-52.2499999999992));
#3989=CARTESIAN_POINT('',(-76.9580463854329,108.363035329266,-39.7047536091873));
#3990=CARTESIAN_POINT('',(-76.9580463854329,108.363035329266,-39.7047536091873));
#3991=CARTESIAN_POINT('',(-73.6123594881249,96.7732359445554,-45.4996533015424));
#3992=CARTESIAN_POINT('Origin',(-69.7150450046476,109.,-52.2499999999992));
#3993=CARTESIAN_POINT('',(-73.6123594881249,96.7732359445554,-45.4996533015424));
#3994=CARTESIAN_POINT('',(-65.8177305211704,96.7732359445554,-59.0003466984559));
#3995=CARTESIAN_POINT('',(-65.8177305211704,96.7732359445554,-59.0003466984559));
#3996=CARTESIAN_POINT('',(-62.4720436238624,108.363035329266,-64.7952463908111));
#3997=CARTESIAN_POINT('Origin',(-69.7150450046476,109.,-52.2499999999992));
#3998=CARTESIAN_POINT('',(-62.4720436238624,108.363035329266,-64.7952463908111));
#3999=CARTESIAN_POINT('',(-66.3693581073396,121.863728726179,-58.0448996923544));
#4000=CARTESIAN_POINT('',(-66.3693581073396,121.863728726179,-58.0448996923544));
#4001=CARTESIAN_POINT('',(-73.0607319019557,121.863728726179,-46.4551003076441));
#4002=CARTESIAN_POINT('Origin',(-69.7150450046476,109.,-52.2499999999992));
#4003=CARTESIAN_POINT('',(-73.0607319019557,121.863728726179,-46.4551003076441));
#4004=CARTESIAN_POINT('Origin',(-63.6528671781565,109.,-48.7499999999993));
#4005=CARTESIAN_POINT('',(-72.1528671781564,109.,-34.0275681356638));
#4006=CARTESIAN_POINT('Origin',(-63.6528671781565,109.,-48.7499999999993));
#4007=CARTESIAN_POINT('',(-56.6032733899647,101.437180526611,-60.9602546138697));
#4008=CARTESIAN_POINT('',(-56.6032733899647,101.437180526611,-60.9602546138697));
#4009=CARTESIAN_POINT('',(-56.8532733899647,100.571155122826,-60.5272419119775));
#4010=CARTESIAN_POINT('',(-56.8532733899647,100.571155122826,-60.5272419119775));
#4011=CARTESIAN_POINT('',(-57.2862860918569,101.071155122826,-59.7772419119775));
#4012=CARTESIAN_POINT('',(-70.4524609663477,100.571155122824,-36.9727580880222));
#4013=CARTESIAN_POINT('',(-70.4524609663477,100.571155122824,-36.9727580880222));
#4014=CARTESIAN_POINT('',(-70.7024609663477,101.437180526609,-36.5397453861299));
#4015=CARTESIAN_POINT('',(-70.7024609663477,101.437180526609,-36.53974538613));
#4016=CARTESIAN_POINT('',(-70.2694482644555,101.937180526609,-37.2897453861299));
#4017=CARTESIAN_POINT('',(-63.9028671781572,124.991664350565,-48.3169872981059));
#4018=CARTESIAN_POINT('',(-63.9028671781572,124.991664350565,-48.3169872981059));
#4019=CARTESIAN_POINT('',(-63.4028671781572,124.991664350565,-49.1830127018903));
#4020=CARTESIAN_POINT('',(-63.4028671781572,124.991664350565,-49.1830127018903));
#4021=CARTESIAN_POINT('',(-63.4028671781572,123.991664350565,-49.1830127018903));
#4022=CARTESIAN_POINT('Origin',(-69.7150450046476,109.,-52.2499999999992));
#4023=CARTESIAN_POINT('',(-78.2150450046475,109.,-37.5275681356637));
#4024=CARTESIAN_POINT('Origin',(-67.1169687932943,109.,-50.7499999999993));
#4025=CARTESIAN_POINT('',(-60.3173750051025,100.571155122826,-62.5272419119774));
#4026=CARTESIAN_POINT('',(-60.7503877069946,101.071155122826,-61.7772419119775));
#4027=CARTESIAN_POINT('',(-60.0673750051025,101.437180526611,-62.9602546138697));
#4028=CARTESIAN_POINT('',(-60.3173750051025,100.571155122826,-62.5272419119774));
#4029=CARTESIAN_POINT('',(-60.0673750051025,101.437180526611,-62.9602546138697));
#4030=CARTESIAN_POINT('',(-66.866968793295,124.991664350565,-51.1830127018903));
#4031=CARTESIAN_POINT('',(-66.866968793295,123.991664350565,-51.1830127018903));
#4032=CARTESIAN_POINT('',(-67.366968793295,124.991664350565,-50.3169872981059));
#4033=CARTESIAN_POINT('',(-66.866968793295,124.991664350565,-51.1830127018903));
#4034=CARTESIAN_POINT('',(-67.366968793295,124.991664350565,-50.3169872981059));
#4035=CARTESIAN_POINT('',(-74.1665625814855,101.437180526609,-38.5397453861299));
#4036=CARTESIAN_POINT('',(-73.7335498795933,101.937180526609,-39.2897453861299));
#4037=CARTESIAN_POINT('',(-73.9165625814855,100.571155122824,-38.9727580880221));
#4038=CARTESIAN_POINT('',(-74.1665625814855,101.437180526609,-38.5397453861299));
#4039=CARTESIAN_POINT('',(-73.9165625814855,100.571155122824,-38.9727580880221));
#4040=CARTESIAN_POINT('',(-73.616968793294,109.,-39.4916697508017));
#4041=CARTESIAN_POINT('Origin',(-67.116968793295,109.,-50.7499999999981));
#4042=CARTESIAN_POINT('Origin',(-119.078493020361,109.,-80.7499999999988));
#4043=CARTESIAN_POINT('',(-122.975807503838,96.7732359445554,-73.9996533015419));
#4044=CARTESIAN_POINT('',(-122.975807503838,96.7732359445554,-73.9996533015419));
#4045=CARTESIAN_POINT('',(-126.321494401146,108.363035329266,-68.2047536091869));
#4046=CARTESIAN_POINT('Origin',(-119.078493020361,109.,-80.7499999999988));
#4047=CARTESIAN_POINT('',(-126.564449609913,108.0824948189,-67.7839428436388));
#4048=CARTESIAN_POINT('',(-122.424179917669,121.863728726179,-74.9551003076436));
#4049=CARTESIAN_POINT('',(-122.424179917669,121.863728726179,-74.9551003076436));
#4050=CARTESIAN_POINT('',(-115.732806123053,121.863728726179,-86.5448996923539));
#4051=CARTESIAN_POINT('Origin',(-119.078493020361,109.,-80.7499999999988));
#4052=CARTESIAN_POINT('',(-115.732806123053,122.42480974691,-86.5448996923539));
#4053=CARTESIAN_POINT('',(-111.835491639576,108.363035329266,-93.2952463908107));
#4054=CARTESIAN_POINT('',(-111.835491639576,108.363035329266,-93.2952463908107));
#4055=CARTESIAN_POINT('',(-115.181178536884,96.7732359445553,-87.5003466984555));
#4056=CARTESIAN_POINT('Origin',(-119.078493020361,109.,-80.7499999999988));
#4057=CARTESIAN_POINT('',(-114.938223328117,96.49269543419,-87.9211574640035));
#4058=CARTESIAN_POINT('Origin',(-75.5607164801933,129.,-55.624999999998));
#4059=CARTESIAN_POINT('',(-75.5607164801933,129.,-59.6249999999981));
#4060=CARTESIAN_POINT('Origin',(-75.5607164801933,129.,-55.624999999998));
#4061=CARTESIAN_POINT('',(-75.5607164801933,129.,-59.1249999999981));
#4062=CARTESIAN_POINT('Origin',(-75.5607164801933,129.,-55.624999999998));
#4063=CARTESIAN_POINT('Origin',(-75.5607164801933,-5.00102499999999,-55.624999999998));
#4064=CARTESIAN_POINT('',(-75.5607164801933,-5.00102499999999,-59.6249999999981));
#4065=CARTESIAN_POINT('',(-77.5607164801934,122.937359864766,-52.1608983848606));
#4066=CARTESIAN_POINT('',(-77.5607164801934,122.937359864766,-52.1608983848601));
#4067=CARTESIAN_POINT('',(-73.5607164801933,122.937359864767,-59.0891016151359));
#4068=CARTESIAN_POINT('Ctrl Pts',(-77.5607164801933,122.937359864766,-52.1608983848601));
#4069=CARTESIAN_POINT('Ctrl Pts',(-77.1232537523542,122.937359864766,-51.9083291611818));
#4070=CARTESIAN_POINT('Ctrl Pts',(-76.60754249421,122.967689419789,-51.7277743724565));
#4071=CARTESIAN_POINT('Ctrl Pts',(-75.5502948880754,123.075440885261,-51.5896430799529));
#4072=CARTESIAN_POINT('Ctrl Pts',(-75.008612000326,123.151115999848,-51.6318312278756));
#4073=CARTESIAN_POINT('Ctrl Pts',(-74.0423701006026,123.291794528869,-51.8907349645996));
#4074=CARTESIAN_POINT('Ctrl Pts',(-73.5520995881099,123.366192507349,-52.1250380084307));
#4075=CARTESIAN_POINT('Ctrl Pts',(-72.7054703736856,123.47098799846,-52.7733608760245));
#4076=CARTESIAN_POINT('Ctrl Pts',(-72.3491310307417,123.5,-53.1876291712969));
#4077=CARTESIAN_POINT('Ctrl Pts',(-71.8440986993692,123.5,-54.0623708286991));
#4078=CARTESIAN_POINT('Ctrl Pts',(-71.6635015031528,123.47098799846,-54.5781038996925));
#4079=CARTESIAN_POINT('Ctrl Pts',(-71.5253520371743,123.366192507349,-55.635467740767));
#4080=CARTESIAN_POINT('Ctrl Pts',(-71.5675749052789,123.29179452887,-56.1772059812275));
#4081=CARTESIAN_POINT('Ctrl Pts',(-71.826478642003,123.151115999849,-57.143447880951));
#4082=CARTESIAN_POINT('Ctrl Pts',(-72.060784078038,123.075440885262,-57.6336530964987));
#4083=CARTESIAN_POINT('Ctrl Pts',(-72.709033089471,122.96768941979,-58.4801907352497));
#4084=CARTESIAN_POINT('Ctrl Pts',(-73.1232537523542,122.937359864767,-58.8365323914576));
#4085=CARTESIAN_POINT('Ctrl Pts',(-73.5607164801933,122.937359864767,-59.0891016151359));
#4086=CARTESIAN_POINT('',(-73.5607164801933,122.937359864767,-59.0891016151359));
#4087=CARTESIAN_POINT('Origin',(-88.2037045535141,128.101020514434,-62.924432567491));
#4088=CARTESIAN_POINT('',(-84.3072367627289,129.005199011952,-62.924432567491));
#4089=CARTESIAN_POINT('Origin',(-88.2037045535141,128.101020514434,-62.924432567491));
#4090=CARTESIAN_POINT('',(-84.7942952365771,128.892176699762,-62.9244325674911));
#4091=CARTESIAN_POINT('Origin',(-88.2037045535141,128.101020514434,-62.9244325674911));
#4092=CARTESIAN_POINT('Origin',(-39.9537393796627,-79.8274313593171,-35.0673021859779));
#4093=CARTESIAN_POINT('',(-36.0572715888775,-78.9232528617992,-35.0673021859779));
#4094=CARTESIAN_POINT('Origin',(-100.711351574804,127.535898384862,-70.1457259421618));
#4095=CARTESIAN_POINT('',(-97.1336428108046,129.324752766862,-70.1457259421618));
#4096=CARTESIAN_POINT('Origin',(-100.711351574804,127.535898384862,-70.1457259421618));
#4097=CARTESIAN_POINT('',(-97.5808564063047,129.101145969112,-70.1457259421618));
#4098=CARTESIAN_POINT('Origin',(-100.711351574804,127.535898384862,-70.1457259421618));
#4099=CARTESIAN_POINT('Origin',(24.6400845185815,-123.166973801907,2.2259594296606));
#4100=CARTESIAN_POINT('',(28.2177932825812,-121.378119419907,2.2259594296606));
#4101=CARTESIAN_POINT('Origin',(-113.529994481957,127.343145750508,-77.5465728752519));
#4102=CARTESIAN_POINT('',(-110.506278697883,129.96176043334,-77.5465728752519));
#4103=CARTESIAN_POINT('Origin',(-113.529994481957,127.343145750508,-77.5465728752519));
#4104=CARTESIAN_POINT('',(-110.884243170892,129.634433597986,-77.5465728752519));
#4105=CARTESIAN_POINT('Origin',(-113.529994481957,127.343145750508,-77.5465728752519));
#4106=CARTESIAN_POINT('Origin',(101.486213576105,-120.9361854544,46.5930927272026));
#4107=CARTESIAN_POINT('',(104.509929360179,-118.317570771568,46.5930927272026));
#4108=CARTESIAN_POINT('Origin',(-75.5607164801933,126.,-55.624999999998));
#4109=CARTESIAN_POINT('',(-75.5607164801933,126.,-59.1249999999981));
#4110=CARTESIAN_POINT('Origin',(-75.5607164801933,126.,-55.624999999998));
#4111=CARTESIAN_POINT('',(-75.5607164801933,126.,-58.4249999999981));
#4112=CARTESIAN_POINT('Origin',(-75.5607164801933,126.,-55.624999999998));
#4113=CARTESIAN_POINT('Origin',(-75.5607164801933,126.,-55.624999999998));
#4114=CARTESIAN_POINT('',(-75.5607164801933,126.,-59.1249999999981));
#4115=CARTESIAN_POINT('Origin',(-87.531272949388,125.203243035567,-62.5362039998373));
#4116=CARTESIAN_POINT('',(-84.121863632451,125.994399220895,-62.5362039998373));
#4117=CARTESIAN_POINT('Origin',(-87.531272949388,125.203243035567,-62.5362039998373));
#4118=CARTESIAN_POINT('',(-84.8037454958384,125.836167983829,-62.5362039998373));
#4119=CARTESIAN_POINT('Origin',(-87.531272949388,125.203243035567,-62.5362039998373));
#4120=CARTESIAN_POINT('Origin',(-87.531272949388,125.203243035567,-62.5362039998373));
#4121=CARTESIAN_POINT('',(-84.121863632451,125.994399220895,-62.5362039998373));
#4122=CARTESIAN_POINT('Origin',(-99.4123134691276,124.937822173509,-69.3957259421618));
#4123=CARTESIAN_POINT('',(-96.281818300628,126.503069757759,-69.3957259421618));
#4124=CARTESIAN_POINT('Origin',(-99.4123134691276,124.937822173509,-69.3957259421618));
#4125=CARTESIAN_POINT('',(-96.907917334328,126.190020240909,-69.3957259421618));
#4126=CARTESIAN_POINT('Origin',(-99.4123134691276,124.937822173509,-69.3957259421618));
#4127=CARTESIAN_POINT('Origin',(-99.4123134691276,124.937822173509,-69.3957259421618));
#4128=CARTESIAN_POINT('',(-96.281818300628,126.503069757759,-69.3957259421618));
#4129=CARTESIAN_POINT('Origin',(-147.457758061401,109.,-97.1347763108453));
#4130=CARTESIAN_POINT('',(-122.114391405223,109.,-67.4916697508013));
#4131=CARTESIAN_POINT('Origin',(-115.614391405224,109.,-78.7499999999976));
#4132=CARTESIAN_POINT('',(-153.9577580614,109.,-85.8764460616489));
#4133=CARTESIAN_POINT('',(-117.386134507203,101.605059126311,-67.4270749801284));
#4134=CARTESIAN_POINT('',(-111.565481622863,103.438089404292,-62.8444992851723));
#4135=CARTESIAN_POINT('Ctrl Pts',(-117.386134507204,101.60505912631,-67.4270749801283));
#4136=CARTESIAN_POINT('Ctrl Pts',(-117.384843998764,101.603815224188,-67.4273233385933));
#4137=CARTESIAN_POINT('Ctrl Pts',(-117.383552105126,101.602572260028,-67.4275705183945));
#4138=CARTESIAN_POINT('Ctrl Pts',(-117.105783250958,101.335811456963,-67.4804062339256));
#4139=CARTESIAN_POINT('Ctrl Pts',(-116.763727423833,101.113949509274,-67.4772489203251));
#4140=CARTESIAN_POINT('Ctrl Pts',(-115.970697123411,100.70633252813,-67.3909870285613));
#4141=CARTESIAN_POINT('Ctrl Pts',(-115.446738163493,100.524469125477,-67.2695400568307));
#4142=CARTESIAN_POINT('Ctrl Pts',(-114.405674258994,100.28486436115,-66.9123137382068));
#4143=CARTESIAN_POINT('Ctrl Pts',(-113.888815670701,100.22768844038,-66.6754382808512));
#4144=CARTESIAN_POINT('Ctrl Pts',(-113.435498258322,100.22768844038,-66.413715350786));
#4145=CARTESIAN_POINT('Ctrl Pts',(-113.045853744828,100.22768844038,-66.1887539860318));
#4146=CARTESIAN_POINT('Ctrl Pts',(-112.64222922698,100.270378061999,-65.9097091373666));
#4147=CARTESIAN_POINT('Ctrl Pts',(-111.934430306435,100.476843984392,-65.2895980494646));
#4148=CARTESIAN_POINT('Ctrl Pts',(-111.630654997402,100.641526829723,-64.9483785209879));
#4149=CARTESIAN_POINT('Ctrl Pts',(-111.2369795781,101.04252635731,-64.3493295404366));
#4150=CARTESIAN_POINT('Ctrl Pts',(-111.099937593526,101.284167988039,-64.0558123049316));
#4151=CARTESIAN_POINT('Ctrl Pts',(-110.986598478824,101.851747702853,-63.5337079966479));
#4152=CARTESIAN_POINT('Ctrl Pts',(-111.009713416376,102.178321465582,-63.3059402798856));
#4153=CARTESIAN_POINT('Ctrl Pts',(-111.191412176548,102.807744434161,-62.9912287955964));
#4154=CARTESIAN_POINT('Ctrl Pts',(-111.351088823113,103.136138059265,-62.8857591987216));
#4155=CARTESIAN_POINT('Ctrl Pts',(-111.565481622863,103.438089404292,-62.8444992851724));
#4156=CARTESIAN_POINT('Ctrl Pts',(-111.565481622863,103.438089404292,-62.8444992851724));
#4157=CARTESIAN_POINT('Ctrl Pts',(-111.575188933326,103.451761204159,-62.8426311124026));
#4158=CARTESIAN_POINT('Ctrl Pts',(-111.585003582125,103.465381199048,-62.8408869585381));
#4159=CARTESIAN_POINT('Ctrl Pts',(-111.823912628857,103.792091077249,-62.8018507603263));
#4160=CARTESIAN_POINT('Ctrl Pts',(-112.112006606371,104.073708899229,-62.8337382694769));
#4161=CARTESIAN_POINT('Ctrl Pts',(-112.759808395975,104.553028941455,-62.9926274651217));
#4162=CARTESIAN_POINT('Ctrl Pts',(-113.170797750173,104.759746443146,-63.1481468200871));
#4163=CARTESIAN_POINT('Ctrl Pts',(-114.013782161377,105.021576797287,-63.5341097697223));
#4164=CARTESIAN_POINT('Ctrl Pts',(-114.445853744829,105.077430701572,-63.7638828554352));
#4165=CARTESIAN_POINT('Ctrl Pts',(-115.288815670702,105.077430701572,-64.2505671502546));
#4166=CARTESIAN_POINT('Ctrl Pts',(-115.767594076423,105.002693000391,-64.5533994185862));
#4167=CARTESIAN_POINT('Ctrl Pts',(-116.652114853179,104.700016463066,-65.1817663880356));
#4168=CARTESIAN_POINT('Ctrl Pts',(-117.058123820432,104.473289105623,-65.5075087398144));
#4169=CARTESIAN_POINT('Ctrl Pts',(-117.59419825037,103.990784840806,-66.0388312545589));
#4170=CARTESIAN_POINT('Ctrl Pts',(-117.798111636135,103.73410733426,-66.281258295277));
#4171=CARTESIAN_POINT('Ctrl Pts',(-117.971447315925,103.296228661322,-66.6204521442011));
#4172=CARTESIAN_POINT('Ctrl Pts',(-118.007599536035,103.14149423203,-66.7297304001928));
#4173=CARTESIAN_POINT('Ctrl Pts',(-118.025761966741,102.824004944285,-66.9316462349407));
#4174=CARTESIAN_POINT('Ctrl Pts',(-118.007691799887,102.661241838733,-67.0242780679549));
#4175=CARTESIAN_POINT('Ctrl Pts',(-117.914598780889,102.338758161266,-67.1855199066884));
#4176=CARTESIAN_POINT('Ctrl Pts',(-117.839876304636,102.180078121956,-67.2536096461054));
#4177=CARTESIAN_POINT('Ctrl Pts',(-117.643713131067,101.879175318306,-67.3610917996573));
#4178=CARTESIAN_POINT('Ctrl Pts',(-117.522786130607,101.736775618063,-67.4007763629426));
#4179=CARTESIAN_POINT('Ctrl Pts',(-117.386134507204,101.60505912631,-67.4270749801282));
#4180=CARTESIAN_POINT('',(-106.165171981646,103.438089404295,-86.8623521842208));
#4181=CARTESIAN_POINT('',(-100.344519097302,101.605059126314,-82.2797764892636));
#4182=CARTESIAN_POINT('Ctrl Pts',(-106.165171981646,103.438089404295,-86.862352184219));
#4183=CARTESIAN_POINT('Ctrl Pts',(-106.14419730415,103.462308875692,-86.8634802540479));
#4184=CARTESIAN_POINT('Ctrl Pts',(-106.12282827633,103.486302635371,-86.8641514184887));
#4185=CARTESIAN_POINT('Ctrl Pts',(-105.818714172361,103.818683816975,-86.8673779259697));
#4186=CARTESIAN_POINT('Ctrl Pts',(-105.472391325601,104.085740432872,-86.7940722130298));
#4187=CARTESIAN_POINT('Ctrl Pts',(-104.731279077633,104.539153956812,-86.5696833263198));
#4188=CARTESIAN_POINT('Ctrl Pts',(-104.271314809741,104.741671619492,-86.3849512882693));
#4189=CARTESIAN_POINT('Ctrl Pts',(-103.33961664048,105.01118751589,-85.9511255373707));
#4190=CARTESIAN_POINT('Ctrl Pts',(-102.867626486497,105.077430701576,-85.7021134546504));
#4191=CARTESIAN_POINT('Ctrl Pts',(-102.441408937237,105.077430701576,-85.4560366378519));
#4192=CARTESIAN_POINT('Ctrl Pts',(-102.014157839508,105.077430701576,-85.2093631015665));
#4193=CARTESIAN_POINT('Ctrl Pts',(-101.56105927878,105.010210941309,-84.9242504184528));
#4194=CARTESIAN_POINT('Ctrl Pts',(-100.752419784988,104.696117862631,-84.3353138424256));
#4195=CARTESIAN_POINT('Ctrl Pts',(-100.397371710978,104.448780822016,-84.0310608152941));
#4196=CARTESIAN_POINT('Ctrl Pts',(-99.9882037851011,103.92339933994,-83.5499074785033));
#4197=CARTESIAN_POINT('Ctrl Pts',(-99.8584603905707,103.660815277971,-83.3448119619325));
#4198=CARTESIAN_POINT('Ctrl Pts',(-99.7452298798465,103.091082457567,-82.9637606339507));
#4199=CARTESIAN_POINT('Ctrl Pts',(-99.7621917782077,102.784236407494,-82.7872192164191));
#4200=CARTESIAN_POINT('Ctrl Pts',(-99.9262957445862,102.215763592511,-82.502982808928));
#4201=CARTESIAN_POINT('Ctrl Pts',(-100.082544658828,101.922589786887,-82.379514298611));
#4202=CARTESIAN_POINT('Ctrl Pts',(-100.312341841756,101.642706629092,-82.2911817419664));
#4203=CARTESIAN_POINT('Ctrl Pts',(-100.328291840436,101.623796748554,-82.2853723510623));
#4204=CARTESIAN_POINT('Ctrl Pts',(-100.344519097301,101.605059126315,-82.2797764892642));
#4205=CARTESIAN_POINT('Ctrl Pts',(-100.344519097301,101.605059126315,-82.2797764892642));
#4206=CARTESIAN_POINT('Ctrl Pts',(-100.550215520806,101.367541355351,-82.2088434432281));
#4207=CARTESIAN_POINT('Ctrl Pts',(-100.802602048525,101.15899254472,-82.1740857015096));
#4208=CARTESIAN_POINT('Ctrl Pts',(-101.47214666584,100.72565116497,-82.1694959867722));
#4209=CARTESIAN_POINT('Ctrl Pts',(-101.955786523501,100.527533200142,-82.2510215111824));
#4210=CARTESIAN_POINT('Ctrl Pts',(-102.926860882229,100.278935400847,-82.5586126482226));
#4211=CARTESIAN_POINT('Ctrl Pts',(-103.414157839508,100.227688440382,-82.784491970971));
#4212=CARTESIAN_POINT('Ctrl Pts',(-104.267626486497,100.227688440382,-83.2772423240549));
#4213=CARTESIAN_POINT('Ctrl Pts',(-104.705846427788,100.278428703028,-83.5847461309404));
#4214=CARTESIAN_POINT('Ctrl Pts',(-105.498304549662,100.491254479672,-84.2597427183605));
#4215=CARTESIAN_POINT('Ctrl Pts',(-105.853076223232,100.653134652889,-84.6266736743588));
#4216=CARTESIAN_POINT('Ctrl Pts',(-106.353797244182,101.032460766724,-85.2674323799564));
#4217=CARTESIAN_POINT('Ctrl Pts',(-106.557061980701,101.260971981571,-85.5885220082683));
#4218=CARTESIAN_POINT('Ctrl Pts',(-106.72625467127,101.679226130855,-86.024626674228));
#4219=CARTESIAN_POINT('Ctrl Pts',(-106.760576424903,101.831187432809,-86.1626137356242));
#4220=CARTESIAN_POINT('Ctrl Pts',(-106.774196861679,102.153837950614,-86.4089088160002));
#4221=CARTESIAN_POINT('Ctrl Pts',(-106.753460724005,102.324558208363,-86.5171780914983));
#4222=CARTESIAN_POINT('Ctrl Pts',(-106.652169358375,102.675441791642,-86.692619883138));
#4223=CARTESIAN_POINT('Ctrl Pts',(-106.572948453007,102.850982888141,-86.7574812847633));
#4224=CARTESIAN_POINT('Ctrl Pts',(-106.38376792248,103.164953280743,-86.8360360636708));
#4225=CARTESIAN_POINT('Ctrl Pts',(-106.28046465974,103.304960886828,-86.8561514599566));
#4226=CARTESIAN_POINT('Ctrl Pts',(-106.165171981646,103.438089404295,-86.862352184219));
#4227=CARTESIAN_POINT('',(-105.707515158216,101.445788778226,-60.813667453584));
#4228=CARTESIAN_POINT('',(-101.324821922316,103.6146594521,-56.8374045514775));
#4229=CARTESIAN_POINT('Ctrl Pts',(-105.707515158216,101.445788778225,-60.8136674535836));
#4230=CARTESIAN_POINT('Ctrl Pts',(-105.483577684551,101.227887906321,-60.8640309956986));
#4231=CARTESIAN_POINT('Ctrl Pts',(-105.222582053125,101.039304544329,-60.8807352012508));
#4232=CARTESIAN_POINT('Ctrl Pts',(-104.602960841079,100.67854055414,-60.8556299182567));
#4233=CARTESIAN_POINT('Ctrl Pts',(-104.1892589951,100.508020898325,-60.7865580098289));
#4234=CARTESIAN_POINT('Ctrl Pts',(-103.362197532696,100.282687776782,-60.5388045693685));
#4235=CARTESIAN_POINT('Ctrl Pts',(-102.949106981883,100.22768844038,-60.359394524506));
#4236=CARTESIAN_POINT('Ctrl Pts',(-102.587887471937,100.22768844038,-60.1508443432025));
#4237=CARTESIAN_POINT('Ctrl Pts',(-102.254878013721,100.22768844038,-59.9585812428588));
#4238=CARTESIAN_POINT('Ctrl Pts',(-101.918162195562,100.275039954704,-59.7132182406853));
#4239=CARTESIAN_POINT('Ctrl Pts',(-101.348088424631,100.488116881772,-59.166211609912));
#4240=CARTESIAN_POINT('Ctrl Pts',(-101.114826914581,100.65473625473,-58.8648160959221));
#4241=CARTESIAN_POINT('Ctrl Pts',(-100.809047976543,101.052694817512,-58.3193334032543));
#4242=CARTESIAN_POINT('Ctrl Pts',(-100.708587237918,101.302215526292,-58.04101395854));
#4243=CARTESIAN_POINT('Ctrl Pts',(-100.646124764096,101.871223563749,-57.5488477901271));
#4244=CARTESIAN_POINT('Ctrl Pts',(-100.683391349424,102.19108472861,-57.3355266127738));
#4245=CARTESIAN_POINT('Ctrl Pts',(-100.861743664517,102.808915271389,-57.0266113413844));
#4246=CARTESIAN_POINT('Ctrl Pts',(-101.013824739271,103.144973641637,-56.9119727511829));
#4247=CARTESIAN_POINT('Ctrl Pts',(-101.251985600091,103.511086021696,-56.8502538040771));
#4248=CARTESIAN_POINT('Ctrl Pts',(-101.287761408094,103.563290529642,-56.8430050519095));
#4249=CARTESIAN_POINT('Ctrl Pts',(-101.324821922315,103.614659452099,-56.8374045514776));
#4250=CARTESIAN_POINT('Ctrl Pts',(-101.324821922315,103.614659452099,-56.8374045514776));
#4251=CARTESIAN_POINT('Ctrl Pts',(-101.507571534895,103.867965453781,-56.8097878465912));
#4252=CARTESIAN_POINT('Ctrl Pts',(-101.722903603191,104.100150075329,-56.8237200261498));
#4253=CARTESIAN_POINT('Ctrl Pts',(-102.23560907329,104.537239540928,-56.9235644528227));
#4254=CARTESIAN_POINT('Ctrl Pts',(-102.577115242381,104.745590666186,-57.0374747177044));
#4255=CARTESIAN_POINT('Ctrl Pts',(-103.286625217418,105.015534918971,-57.3429707585513));
#4256=CARTESIAN_POINT('Ctrl Pts',(-103.654878013722,105.077430701572,-57.5337101122621));
#4257=CARTESIAN_POINT('Ctrl Pts',(-104.349106981883,105.077430701572,-57.9345233939092));
#4258=CARTESIAN_POINT('Ctrl Pts',(-104.725589216724,105.005615111484,-58.1773409020166));
#4259=CARTESIAN_POINT('Ctrl Pts',(-105.40533608587,104.720635512592,-58.6802507026948));
#4260=CARTESIAN_POINT('Ctrl Pts',(-105.708442531058,104.5080414619,-58.9408794643765));
#4261=CARTESIAN_POINT('Ctrl Pts',(-106.134628803274,104.039966782051,-59.3986735814598));
#4262=CARTESIAN_POINT('Ctrl Pts',(-106.301658407902,103.762601478164,-59.628755601445));
#4263=CARTESIAN_POINT('Ctrl Pts',(-106.466981515918,103.150363245665,-60.0574871392715));
#4264=CARTESIAN_POINT('Ctrl Pts',(-106.463597321879,102.815336528851,-60.256562220115));
#4265=CARTESIAN_POINT('Ctrl Pts',(-106.281537692062,102.184663471148,-60.5718987489666));
#4266=CARTESIAN_POINT('Ctrl Pts',(-106.096327018674,101.866378403104,-60.6994795605523));
#4267=CARTESIAN_POINT('Ctrl Pts',(-105.801011946827,101.53963142162,-60.790807331965));
#4268=CARTESIAN_POINT('Ctrl Pts',(-105.755075673419,101.492067221763,-60.8029710928037));
#4269=CARTESIAN_POINT('Ctrl Pts',(-105.707515158216,101.445788778225,-60.8136674535836));
#4270=CARTESIAN_POINT('',(-94.501534612098,103.614659452104,-80.2229951080884));
#4271=CARTESIAN_POINT('',(-90.1188413761952,101.445788778232,-76.2467322059816));
#4272=CARTESIAN_POINT('Ctrl Pts',(-94.5015346120983,103.614659452105,-80.222995108087));
#4273=CARTESIAN_POINT('Ctrl Pts',(-94.2999319259417,103.85835031517,-80.2346736634614));
#4274=CARTESIAN_POINT('Ctrl Pts',(-94.0660003649607,104.078184573876,-80.204501523942));
#4275=CARTESIAN_POINT('Ctrl Pts',(-93.506215357663,104.508041461903,-80.0757568941915));
#4276=CARTESIAN_POINT('Ctrl Pts',(-93.1289510064958,104.720635512595,-79.9435733934488));
#4277=CARTESIAN_POINT('Ctrl Pts',(-92.353544908723,105.005615111488,-79.6063502369639));
#4278=CARTESIAN_POINT('Ctrl Pts',(-91.9550176607982,105.077430701576,-79.4017158115723));
#4279=CARTESIAN_POINT('Ctrl Pts',(-91.5937981508529,105.077430701576,-79.1931656302689));
#4280=CARTESIAN_POINT('Ctrl Pts',(-91.2445310553966,105.077430701576,-78.9915161786881));
#4281=CARTESIAN_POINT('Ctrl Pts',(-90.8794457263923,105.009294935457,-78.75672916701));
#4282=CARTESIAN_POINT('Ctrl Pts',(-90.2394279750154,104.71379978534,-78.2726325195484));
#4283=CARTESIAN_POINT('Ctrl Pts',(-89.9651725619102,104.486205632632,-78.0225716794456));
#4284=CARTESIAN_POINT('Ctrl Pts',(-89.615152325688,103.992202355958,-77.5948073108704));
#4285=CARTESIAN_POINT('Ctrl Pts',(-89.4966157452444,103.711875068197,-77.3893068873646));
#4286=CARTESIAN_POINT('Ctrl Pts',(-89.4038756583846,103.11192693574,-77.0059525649689));
#4287=CARTESIAN_POINT('Ctrl Pts',(-89.4297352858526,102.792723417415,-76.8274306857825));
#4288=CARTESIAN_POINT('Ctrl Pts',(-89.5987392296941,102.207276582589,-76.5347072683697));
#4289=CARTESIAN_POINT('Ctrl Pts',(-89.7529823542094,101.902585866878,-76.4012820305381));
#4290=CARTESIAN_POINT('Ctrl Pts',(-90.0135013341837,101.566233275656,-76.2843454877329));
#4291=CARTESIAN_POINT('Ctrl Pts',(-90.0649390949408,101.505064596095,-76.2644831614807));
#4292=CARTESIAN_POINT('Ctrl Pts',(-90.1188413761922,101.445788778236,-76.2467322059833));
#4293=CARTESIAN_POINT('Ctrl Pts',(-90.1188413761922,101.445788778236,-76.2467322059833));
#4294=CARTESIAN_POINT('Ctrl Pts',(-90.3002565105157,101.246288307949,-76.1869890578052));
#4295=CARTESIAN_POINT('Ctrl Pts',(-90.5105127919593,101.068816696773,-76.1519939958911));
#4296=CARTESIAN_POINT('Ctrl Pts',(-91.0593017712658,100.696030871333,-76.1274842987972));
#4297=CARTESIAN_POINT('Ctrl Pts',(-91.4519661767371,100.513444242339,-76.1724547480489));
#4298=CARTESIAN_POINT('Ctrl Pts',(-92.2447448611874,100.279759997467,-76.3919616980159));
#4299=CARTESIAN_POINT('Ctrl Pts',(-92.6445310553966,100.227688440383,-76.5666450480926));
#4300=CARTESIAN_POINT('Ctrl Pts',(-93.3550176607982,100.227688440383,-76.9768446809768));
#4301=CARTESIAN_POINT('Ctrl Pts',(-93.7169365927499,100.282687776784,-77.2448865696132));
#4302=CARTESIAN_POINT('Ctrl Pts',(-94.3450280972656,100.508020898327,-77.8372660863158));
#4303=CARTESIAN_POINT('Ctrl Pts',(-94.6116970476415,100.678540554143,-78.1610064403122));
#4304=CARTESIAN_POINT('Ctrl Pts',(-94.9727271872904,101.071379412638,-78.7316542894256));
#4305=CARTESIAN_POINT('Ctrl Pts',(-95.1064606462321,101.310297639174,-79.0194069254365));
#4306=CARTESIAN_POINT('Ctrl Pts',(-95.2231499598568,101.866378403107,-79.5323746661135));
#4307=CARTESIAN_POINT('Ctrl Pts',(-95.2052670726821,102.184663471151,-79.7565622201121));
#4308=CARTESIAN_POINT('Ctrl Pts',(-95.0232074428643,102.815336528854,-80.0718987489636));
#4309=CARTESIAN_POINT('Ctrl Pts',(-94.8524954626127,103.150363245668,-80.174367087394));
#4310=CARTESIAN_POINT('Ctrl Pts',(-94.5857570770073,103.510107742139,-80.2161985863255));
#4311=CARTESIAN_POINT('Ctrl Pts',(-94.5443515978532,103.562903652559,-80.2205147813183));
#4312=CARTESIAN_POINT('Ctrl Pts',(-94.5015346120983,103.614659452105,-80.222995108087));
#4313=CARTESIAN_POINT('',(-94.2209929096256,101.354811290699,-54.2576156201439));
#4314=CARTESIAN_POINT('',(-90.5178421019398,103.716919354992,-50.5448617949466));
#4315=CARTESIAN_POINT('Ctrl Pts',(-94.2209929096261,101.354811290699,-54.2576156201434));
#4316=CARTESIAN_POINT('Ctrl Pts',(-94.0304505856294,101.165865871972,-54.3062458592498));
#4317=CARTESIAN_POINT('Ctrl Pts',(-93.8147279386984,100.999081132478,-54.3308652529223));
#4318=CARTESIAN_POINT('Ctrl Pts',(-93.2853347608051,100.664686636251,-54.335231850713));
#4319=CARTESIAN_POINT('Ctrl Pts',(-92.9240531847944,100.499668449628,-54.2909952556545));
#4320=CARTESIAN_POINT('Ctrl Pts',(-92.1976667058189,100.281331189612,-54.0944571890166));
#4321=CARTESIAN_POINT('Ctrl Pts',(-91.8328571384615,100.22768844038,-53.9414246850278));
#4322=CARTESIAN_POINT('Ctrl Pts',(-91.5141993333915,100.22768844038,-53.7574475154913));
#4323=CARTESIAN_POINT('Ctrl Pts',(-91.1998056536407,100.22768844038,-53.5759322398556));
#4324=CARTESIAN_POINT('Ctrl Pts',(-90.8886903708508,100.280334555034,-53.3396967948896));
#4325=CARTESIAN_POINT('Ctrl Pts',(-90.3733823362884,100.504055421459,-52.8139276391242));
#4326=CARTESIAN_POINT('Ctrl Pts',(-90.1688519647511,100.67573731595,-52.5249835715961));
#4327=CARTESIAN_POINT('Ctrl Pts',(-89.9037680431757,101.07557755986,-52.0026890248464));
#4328=CARTESIAN_POINT('Ctrl Pts',(-89.8203132445372,101.325643828305,-51.7350194741849));
#4329=CARTESIAN_POINT('Ctrl Pts',(-89.7787639540569,101.887795138889,-51.2622217134503));
#4330=CARTESIAN_POINT('Ctrl Pts',(-89.8201747804601,102.200227598979,-51.0575503555047));
#4331=CARTESIAN_POINT('Ctrl Pts',(-89.9932484568848,102.799772401019,-50.7577779544845));
#4332=CARTESIAN_POINT('Ctrl Pts',(-90.1366138563365,103.127423563352,-50.6424075012184));
#4333=CARTESIAN_POINT('Ctrl Pts',(-90.3868899039983,103.531966317969,-50.5657018885759));
#4334=CARTESIAN_POINT('Ctrl Pts',(-90.4505284239739,103.625948972014,-50.5527189917843));
#4335=CARTESIAN_POINT('Ctrl Pts',(-90.5178421019398,103.716919354992,-50.5448617949466));
#4336=CARTESIAN_POINT('Ctrl Pts',(-90.5178421019398,103.716919354992,-50.5448617949466));
#4337=CARTESIAN_POINT('Ctrl Pts',(-90.6677586076694,103.919522486378,-50.5273627734945));
#4338=CARTESIAN_POINT('Ctrl Pts',(-90.8363800498654,104.106877932436,-50.5357972502939));
#4339=CARTESIAN_POINT('Ctrl Pts',(-91.2761732604758,104.511610804944,-50.6070468270981));
#4340=CARTESIAN_POINT('Ctrl Pts',(-91.5920360022583,104.725595554037,-50.7031575728346));
#4341=CARTESIAN_POINT('Ctrl Pts',(-92.2536368706955,105.008647929721,-50.9755401075456));
#4342=CARTESIAN_POINT('Ctrl Pts',(-92.5998056536411,105.077430701572,-51.1510611092587));
#4343=CARTESIAN_POINT('Ctrl Pts',(-93.232857138462,105.077430701572,-51.5165535544309));
#4344=CARTESIAN_POINT('Ctrl Pts',(-93.5619700271323,105.00741652851,-51.7314145195672));
#4345=CARTESIAN_POINT('Ctrl Pts',(-94.1455671289826,104.731116876602,-52.1752710421669));
#4346=CARTESIAN_POINT('Ctrl Pts',(-94.3998110409153,104.525345718212,-52.4049023097321));
#4347=CARTESIAN_POINT('Ctrl Pts',(-94.768377540354,104.0613168212,-52.8259509372149));
#4348=CARTESIAN_POINT('Ctrl Pts',(-94.9105232806575,103.7725092302,-53.0468145506106));
#4349=CARTESIAN_POINT('Ctrl Pts',(-95.0354212815802,103.14720818058,-53.4590643079669));
#4350=CARTESIAN_POINT('Ctrl Pts',(-95.0172814114049,102.810893242388,-53.6509908389482));
#4351=CARTESIAN_POINT('Ctrl Pts',(-94.8377871142222,102.18910675761,-53.9618840813374));
#4352=CARTESIAN_POINT('Ctrl Pts',(-94.66647754768,101.869149596082,-54.0980936002161));
#4353=CARTESIAN_POINT('Ctrl Pts',(-94.365959399355,101.505588017214,-54.2160961273275));
#4354=CARTESIAN_POINT('Ctrl Pts',(-94.2953494579818,101.428544668509,-54.238638331267));
#4355=CARTESIAN_POINT('Ctrl Pts',(-94.2209929096261,101.354811290699,-54.2576156201434));
#4356=CARTESIAN_POINT('',(-83.0247832218288,103.716919354995,-73.6500196516034));
#4357=CARTESIAN_POINT('',(-79.3216324141422,101.354811290702,-69.9372658264059));
#4358=CARTESIAN_POINT('Ctrl Pts',(-83.0247832218292,103.716919354995,-73.6500196516021));
#4359=CARTESIAN_POINT('Ctrl Pts',(-82.8561874835582,103.929460895585,-73.6618384029087));
#4360=CARTESIAN_POINT('Ctrl Pts',(-82.6660644120803,104.123947093647,-73.6439402061671));
#4361=CARTESIAN_POINT('Ctrl Pts',(-82.1939330584629,104.523769595123,-73.5508930043753));
#4362=CARTESIAN_POINT('Ctrl Pts',(-81.8675496354975,104.73010984644,-73.445550762439));
#4363=CARTESIAN_POINT('Ctrl Pts',(-81.1904340361545,105.007198663853,-73.1618575252943));
#4364=CARTESIAN_POINT('Ctrl Pts',(-80.8392691645201,105.077430701576,-72.9840354250022));
#4365=CARTESIAN_POINT('Ctrl Pts',(-80.5201100123077,105.077430701576,-72.799768802558));
#4366=CARTESIAN_POINT('Ctrl Pts',(-80.2107074631239,105.077430701576,-72.6211351574988));
#4367=CARTESIAN_POINT('Ctrl Pts',(-79.8902928105569,105.010817414927,-72.4125520697033));
#4368=CARTESIAN_POINT('Ctrl Pts',(-79.3296459208272,104.735983399352,-71.9826313276384));
#4369=CARTESIAN_POINT('Ctrl Pts',(-79.0898300656876,104.528017888669,-71.760587957699));
#4370=CARTESIAN_POINT('Ctrl Pts',(-78.7510680657571,104.056494164301,-71.353383279585));
#4371=CARTESIAN_POINT('Ctrl Pts',(-78.6282785579301,103.763711210128,-71.1414137376349));
#4372=CARTESIAN_POINT('Ctrl Pts',(-78.5328756547392,103.137634877854,-70.745080894813));
#4373=CARTESIAN_POINT('Ctrl Pts',(-78.5604078289852,102.804749283705,-70.5600387968433));
#4374=CARTESIAN_POINT('Ctrl Pts',(-78.7363549099663,102.1952507163,-70.2552895131407));
#4375=CARTESIAN_POINT('Ctrl Pts',(-78.8964707374473,101.878104564589,-70.1153157381806));
#4376=CARTESIAN_POINT('Ctrl Pts',(-79.1804605765672,101.511189981574,-69.9855724361914));
#4377=CARTESIAN_POINT('Ctrl Pts',(-79.2490780626133,101.431324815456,-69.9596178450133));
#4378=CARTESIAN_POINT('Ctrl Pts',(-79.3216324141422,101.354811290702,-69.9372658264059));
#4379=CARTESIAN_POINT('Ctrl Pts',(-79.3216324141422,101.354811290702,-69.9372658264059));
#4380=CARTESIAN_POINT('Ctrl Pts',(-79.4994951487113,101.167242875335,-69.8824711646265));
#4381=CARTESIAN_POINT('Ctrl Pts',(-79.7016131069151,101.000214480644,-69.8498916678611));
#4382=CARTESIAN_POINT('Ctrl Pts',(-80.2057230797504,100.662451096332,-69.8278045615312));
#4383=CARTESIAN_POINT('Ctrl Pts',(-80.5536874604562,100.495779124926,-69.8625291904263));
#4384=CARTESIAN_POINT('Ctrl Pts',(-81.2563406796862,100.27868878512,-70.0464877548005));
#4385=CARTESIAN_POINT('Ctrl Pts',(-81.6107074631236,100.227688440383,-70.1962640269031));
#4386=CARTESIAN_POINT('Ctrl Pts',(-82.2392691645199,100.227688440383,-70.5591642944065));
#4387=CARTESIAN_POINT('Ctrl Pts',(-82.5546266768382,100.281496733901,-70.7990065603189));
#4388=CARTESIAN_POINT('Ctrl Pts',(-83.0885412363331,100.500470869914,-71.330731274177));
#4389=CARTESIAN_POINT('Ctrl Pts',(-83.3075860460983,100.665962481951,-71.6219894477902));
#4390=CARTESIAN_POINT('Ctrl Pts',(-83.6098374691532,101.054698410516,-72.1567503717173));
#4391=CARTESIAN_POINT('Ctrl Pts',(-83.7166215744316,101.303006298545,-72.4375565865388));
#4392=CARTESIAN_POINT('Ctrl Pts',(-83.7911705443989,101.870113330836,-72.9351916366745));
#4393=CARTESIAN_POINT('Ctrl Pts',(-83.7588055350932,102.189611224737,-73.1512430725076));
#4394=CARTESIAN_POINT('Ctrl Pts',(-83.5796024921405,102.810388775268,-73.4616318477727));
#4395=CARTESIAN_POINT('Ctrl Pts',(-83.4227987210069,103.14619075922,-73.5732303508662));
#4396=CARTESIAN_POINT('Ctrl Pts',(-83.1543827768569,103.546695163547,-73.6361875753525));
#4397=CARTESIAN_POINT('Ctrl Pts',(-83.0912106178557,103.633177136873,-73.6453630162586));
#4398=CARTESIAN_POINT('Ctrl Pts',(-83.0247832218292,103.716919354995,-73.6500196516021));
#4399=CARTESIAN_POINT('',(-79.2724338250639,100.514077983564,-46.3961169753473));
#4400=CARTESIAN_POINT('',(-82.9097405209592,104.714077983563,-45.6961169753459));
#4401=CARTESIAN_POINT('Ctrl Pts',(-79.2724338250643,100.514077983563,-46.3961169753468));
#4402=CARTESIAN_POINT('Ctrl Pts',(-79.1265511423845,100.610404906306,-46.2160498567682));
#4403=CARTESIAN_POINT('Ctrl Pts',(-79.0063377502804,100.729412390803,-46.0312428512855));
#4404=CARTESIAN_POINT('Ctrl Pts',(-78.7783882480642,101.056823805357,-45.5960981587349));
#4405=CARTESIAN_POINT('Ctrl Pts',(-78.6879980806413,101.308592332844,-45.3220312346838));
#4406=CARTESIAN_POINT('Ctrl Pts',(-78.637346637553,101.87720020589,-44.8375673373119));
#4407=CARTESIAN_POINT('Ctrl Pts',(-78.6768221832288,102.194506798829,-44.627746600585));
#4408=CARTESIAN_POINT('Ctrl Pts',(-78.8531987651598,102.805493201169,-44.3222533994151));
#4409=CARTESIAN_POINT('Ctrl Pts',(-79.001482969892,103.138605462875,-44.2068647088189));
#4410=CARTESIAN_POINT('Ctrl Pts',(-79.3969069246043,103.764324604201,-44.094165099005));
#4411=CARTESIAN_POINT('Ctrl Pts',(-79.6443545210792,104.056618970362,-44.0962005762319));
#4412=CARTESIAN_POINT('Ctrl Pts',(-80.1647562293486,104.52433820779,-44.1867417540882));
#4413=CARTESIAN_POINT('Ctrl Pts',(-80.4728761101798,104.731264722065,-44.2812762970742));
#4414=CARTESIAN_POINT('Ctrl Pts',(-81.1163900166925,105.008060588784,-44.5457120366282));
#4415=CARTESIAN_POINT('Ctrl Pts',(-81.4522447708355,105.077430701572,-44.7150138327633));
#4416=CARTESIAN_POINT('Ctrl Pts',(-82.0632775106341,105.077430701572,-45.0677937495697));
#4417=CARTESIAN_POINT('Ctrl Pts',(-82.3778245440648,105.008060588784,-45.2740016005717));
#4418=CARTESIAN_POINT('Ctrl Pts',(-82.7431217757092,104.824474558593,-45.5559387185791));
#4419=CARTESIAN_POINT('Ctrl Pts',(-82.8290587463787,104.772275635182,-45.6260680866036));
#4420=CARTESIAN_POINT('Ctrl Pts',(-82.9097405209591,104.714077983563,-45.6961169753458));
#4421=CARTESIAN_POINT('Ctrl Pts',(-82.9097405209591,104.714077983563,-45.6961169753458));
#4422=CARTESIAN_POINT('Ctrl Pts',(-83.0761634408585,104.594033237844,-45.8406073594606));
#4423=CARTESIAN_POINT('Ctrl Pts',(-83.2198007296756,104.447978167203,-45.9848429857255));
#4424=CARTESIAN_POINT('Ctrl Pts',(-83.5031306358671,104.056618970362,-46.3240660048471));
#4425=CARTESIAN_POINT('Ctrl Pts',(-83.6286172090919,103.764324604201,-46.5373441708864));
#4426=CARTESIAN_POINT('Ctrl Pts',(-83.7287284613526,103.138605462875,-46.936141165839));
#4427=CARTESIAN_POINT('Ctrl Pts',(-83.7029410263529,102.805493201169,-47.1222533994152));
#4428=CARTESIAN_POINT('Ctrl Pts',(-83.5265644444219,102.194506798829,-47.427746600585));
#4429=CARTESIAN_POINT('Ctrl Pts',(-83.3645921290135,101.87720020589,-47.5668437943321));
#4430=CARTESIAN_POINT('Ctrl Pts',(-82.9197083651289,101.308592332844,-47.7652103065652));
#4431=CARTESIAN_POINT('Ctrl Pts',(-82.6371643628521,101.056823805357,-47.8239635873502));
#4432=CARTESIAN_POINT('Ctrl Pts',(-82.0505767043741,100.665529520269,-47.8480598380025));
#4433=CARTESIAN_POINT('Ctrl Pts',(-81.7069979829943,100.499547348265,-47.8149418084238));
#4434=CARTESIAN_POINT('Ctrl Pts',(-81.0131896142114,100.280826524207,-47.637618632861));
#4435=CARTESIAN_POINT('Ctrl Pts',(-80.6632775106336,100.227688440379,-47.4926648801669));
#4436=CARTESIAN_POINT('Ctrl Pts',(-80.3577611407344,100.227688440379,-47.3162749217637));
#4437=CARTESIAN_POINT('Ctrl Pts',(-80.0522447708351,100.227688440379,-47.1398849633606));
#4438=CARTESIAN_POINT('Ctrl Pts',(-79.7517550868392,100.280826524207,-46.9093290689175));
#4439=CARTESIAN_POINT('Ctrl Pts',(-79.4198158701761,100.42589403654,-46.5696141741228));
#4440=CARTESIAN_POINT('Ctrl Pts',(-79.3431576996741,100.467378724402,-46.4834134527748));
#4441=CARTESIAN_POINT('Ctrl Pts',(-79.2724338250643,100.514077983563,-46.3961169753468));
#4442=CARTESIAN_POINT('',(-68.2116924394259,104.714077983566,-65.5538830246524));
#4443=CARTESIAN_POINT('',(-71.8489991353209,100.514077983566,-64.8538830246516));
#4444=CARTESIAN_POINT('Ctrl Pts',(-68.2116924394265,104.714077983567,-65.5538830246511));
#4445=CARTESIAN_POINT('Ctrl Pts',(-68.0452695195272,104.594033237848,-65.4093926405365));
#4446=CARTESIAN_POINT('Ctrl Pts',(-67.9016322307103,104.447978167207,-65.2651570142717));
#4447=CARTESIAN_POINT('Ctrl Pts',(-67.6183023245187,104.056618970366,-64.9259339951503));
#4448=CARTESIAN_POINT('Ctrl Pts',(-67.4928157512939,103.764324604205,-64.7126558291111));
#4449=CARTESIAN_POINT('Ctrl Pts',(-67.3927044990331,103.138605462879,-64.3138588341587));
#4450=CARTESIAN_POINT('Ctrl Pts',(-67.4184919340327,102.805493201172,-64.1277466005826));
#4451=CARTESIAN_POINT('Ctrl Pts',(-67.5948685159636,102.194506798833,-63.8222533994129));
#4452=CARTESIAN_POINT('Ctrl Pts',(-67.7568408313719,101.877200205893,-63.683156205666));
#4453=CARTESIAN_POINT('Ctrl Pts',(-68.2017245952565,101.308592332847,-63.484789693433));
#4454=CARTESIAN_POINT('Ctrl Pts',(-68.4842685975332,101.056823805361,-63.4260364126481));
#4455=CARTESIAN_POINT('Ctrl Pts',(-69.0708562560112,100.665529520272,-63.4019401619959));
#4456=CARTESIAN_POINT('Ctrl Pts',(-69.4144349773908,100.499547348269,-63.4350581915746));
#4457=CARTESIAN_POINT('Ctrl Pts',(-70.1082433461736,100.28082652421,-63.6123813671375));
#4458=CARTESIAN_POINT('Ctrl Pts',(-70.4581554497515,100.227688440383,-63.7573351198316));
#4459=CARTESIAN_POINT('Ctrl Pts',(-71.0691881895501,100.227688440383,-64.110115036638));
#4460=CARTESIAN_POINT('Ctrl Pts',(-71.369677873546,100.28082652421,-64.340670931081));
#4461=CARTESIAN_POINT('Ctrl Pts',(-71.701617090209,100.425894036543,-64.6803858258755));
#4462=CARTESIAN_POINT('Ctrl Pts',(-71.7782752607111,100.467378724405,-64.7665865472236));
#4463=CARTESIAN_POINT('Ctrl Pts',(-71.8489991353208,100.514077983566,-64.8538830246515));
#4464=CARTESIAN_POINT('Ctrl Pts',(-71.8489991353208,100.514077983566,-64.8538830246515));
#4465=CARTESIAN_POINT('Ctrl Pts',(-71.9948818180007,100.61040490631,-65.0339501432301));
#4466=CARTESIAN_POINT('Ctrl Pts',(-72.1150952101049,100.729412390806,-65.2187571487129));
#4467=CARTESIAN_POINT('Ctrl Pts',(-72.3430447123212,101.056823805361,-65.6539018412633));
#4468=CARTESIAN_POINT('Ctrl Pts',(-72.4334348797441,101.308592332847,-65.9279687653144));
#4469=CARTESIAN_POINT('Ctrl Pts',(-72.4840863228325,101.877200205893,-66.4124326626861));
#4470=CARTESIAN_POINT('Ctrl Pts',(-72.4446107771567,102.194506798833,-66.622253399413));
#4471=CARTESIAN_POINT('Ctrl Pts',(-72.2682341952258,102.805493201172,-66.9277466005826));
#4472=CARTESIAN_POINT('Ctrl Pts',(-72.1199499904937,103.138605462879,-67.0431352911788));
#4473=CARTESIAN_POINT('Ctrl Pts',(-71.7245260357815,103.764324604205,-67.1558349009925));
#4474=CARTESIAN_POINT('Ctrl Pts',(-71.4770784393067,104.056618970366,-67.1537994237656));
#4475=CARTESIAN_POINT('Ctrl Pts',(-70.9566767310373,104.524338207794,-67.0632582459091));
#4476=CARTESIAN_POINT('Ctrl Pts',(-70.6485568502061,104.731264722069,-66.968723702923));
#4477=CARTESIAN_POINT('Ctrl Pts',(-70.0050429436934,105.008060588788,-66.7042879633689));
#4478=CARTESIAN_POINT('Ctrl Pts',(-69.6691881895505,105.077430701576,-66.5349861672338));
#4479=CARTESIAN_POINT('Ctrl Pts',(-69.3636718196512,105.077430701576,-66.3585962088306));
#4480=CARTESIAN_POINT('Ctrl Pts',(-69.0581554497519,105.077430701576,-66.1822062504275));
#4481=CARTESIAN_POINT('Ctrl Pts',(-68.7436084163211,105.008060588788,-65.9759983994254));
#4482=CARTESIAN_POINT('Ctrl Pts',(-68.3783111846766,104.824474558597,-65.694061281418));
#4483=CARTESIAN_POINT('Ctrl Pts',(-68.292374214007,104.772275635186,-65.6239319133934));
#4484=CARTESIAN_POINT('Ctrl Pts',(-68.2116924394265,104.714077983567,-65.5538830246511));
#4485=CARTESIAN_POINT('',(-112.569378637745,121.956851469395,-75.7699408736866));
#4486=CARTESIAN_POINT('',(-105.161274966764,121.956851469395,-73.9369105957041));
#4487=CARTESIAN_POINT('Ctrl Pts',(-112.569378637745,121.956851469395,-75.7699408736867));
#4488=CARTESIAN_POINT('Ctrl Pts',(-112.569272008943,121.95672834506,-75.7681386924676));
#4489=CARTESIAN_POINT('Ctrl Pts',(-112.569163342679,121.956605035935,-75.7663364623398));
#4490=CARTESIAN_POINT('Ctrl Pts',(-112.545386428826,121.930081208774,-75.3792452325324));
#4491=CARTESIAN_POINT('Ctrl Pts',(-112.425619842949,121.895265649918,-74.9910716591131));
#4492=CARTESIAN_POINT('Ctrl Pts',(-112.050450493293,121.820378366244,-74.1810533701236));
#4493=CARTESIAN_POINT('Ctrl Pts',(-111.722843184654,121.775514411454,-73.719515362228));
#4494=CARTESIAN_POINT('Ctrl Pts',(-110.943904850608,121.712442638456,-72.9082742376171));
#4495=CARTESIAN_POINT('Ctrl Pts',(-110.491771010159,121.694880858045,-72.5592922284894));
#4496=CARTESIAN_POINT('Ctrl Pts',(-110.03845359778,121.694880858045,-72.2975692984242));
#4497=CARTESIAN_POINT('Ctrl Pts',(-109.648809084286,121.694880858045,-72.07260793367));
#4498=CARTESIAN_POINT('Ctrl Pts',(-109.196813666427,121.708045140711,-71.8773439414328));
#4499=CARTESIAN_POINT('Ctrl Pts',(-108.262263007713,121.76340957246,-71.6499783847423));
#4500=CARTESIAN_POINT('Ctrl Pts',(-107.779465090809,121.805444228819,-71.6188351088017));
#4501=CARTESIAN_POINT('Ctrl Pts',(-106.970686338396,121.883764743458,-71.7387661915901));
#4502=CARTESIAN_POINT('Ctrl Pts',(-106.589756165829,121.923740934709,-71.8676756890549));
#4503=CARTESIAN_POINT('Ctrl Pts',(-105.93403329749,121.982452032228,-72.2850075992705));
#4504=CARTESIAN_POINT('Ctrl Pts',(-105.659130074434,121.999999999998,-72.5734224782579));
#4505=CARTESIAN_POINT('Ctrl Pts',(-105.295732554092,121.999999999998,-73.2028454468363));
#4506=CARTESIAN_POINT('Ctrl Pts',(-105.184827334639,121.984047401261,-73.5660373895111));
#4507=CARTESIAN_POINT('Ctrl Pts',(-105.161274966764,121.956851469395,-73.936910595704));
#4508=CARTESIAN_POINT('Ctrl Pts',(-105.161274966764,121.956851469395,-73.936910595704));
#4509=CARTESIAN_POINT('Ctrl Pts',(-105.160208558995,121.955620087771,-73.9537030502982));
#4510=CARTESIAN_POINT('Ctrl Pts',(-105.159312222542,121.954368073319,-73.9705108670905));
#4511=CARTESIAN_POINT('Ctrl Pts',(-105.141806095166,121.923740934709,-74.3755987782653));
#4512=CARTESIAN_POINT('Ctrl Pts',(-105.220632281856,121.883764743458,-74.7699487335092));
#4513=CARTESIAN_POINT('Ctrl Pts',(-105.521158293664,121.805444228818,-75.5303372205339));
#4514=CARTESIAN_POINT('Ctrl Pts',(-105.789528120238,121.763409572459,-75.9328808434969));
#4515=CARTESIAN_POINT('Ctrl Pts',(-106.453707797634,121.708045140711,-76.628542676721));
#4516=CARTESIAN_POINT('Ctrl Pts',(-106.848809084286,121.694880858045,-76.9223501948628));
#4517=CARTESIAN_POINT('Ctrl Pts',(-107.691771010159,121.694880858045,-77.4090344896822));
#4518=CARTESIAN_POINT('Ctrl Pts',(-108.220065215752,121.712442638456,-77.6261028768581));
#4519=CARTESIAN_POINT('Ctrl Pts',(-109.312089805283,121.775514411454,-77.895062699818));
#4520=CARTESIAN_POINT('Ctrl Pts',(-109.875597099252,121.820378366244,-77.948009947617));
#4521=CARTESIAN_POINT('Ctrl Pts',(-110.764678189875,121.895265649918,-77.8679069906454));
#4522=CARTESIAN_POINT('Ctrl Pts',(-111.160729658472,121.930081208774,-77.7775411098295));
#4523=CARTESIAN_POINT('Ctrl Pts',(-111.678984353092,121.96968170959,-77.5193177005707));
#4524=CARTESIAN_POINT('Ctrl Pts',(-111.839559773292,121.980744602752,-77.4130886523666));
#4525=CARTESIAN_POINT('Ctrl Pts',(-112.11953636853,121.995916933756,-77.161529052004));
#4526=CARTESIAN_POINT('Ctrl Pts',(-112.238887146792,121.999999999998,-77.016140826053));
#4527=CARTESIAN_POINT('Ctrl Pts',(-112.425073184787,121.999999999998,-76.693657148586));
#4528=CARTESIAN_POINT('Ctrl Pts',(-112.491307692741,121.995916933756,-76.5176022296746));
#4529=CARTESIAN_POINT('Ctrl Pts',(-112.568812151847,121.980815574618,-76.1510781390455));
#4530=CARTESIAN_POINT('Ctrl Pts',(-112.580669535468,121.969889075075,-75.9607734026514));
#4531=CARTESIAN_POINT('Ctrl Pts',(-112.569378637745,121.956851469395,-75.7699408736867));
#4532=CARTESIAN_POINT('',(-101.043673435707,121.93955176967,-68.8916782754278));
#4533=CARTESIAN_POINT('',(-94.7826830987082,121.939551769669,-68.1687213841338));
#4534=CARTESIAN_POINT('Ctrl Pts',(-101.043673435707,121.93955176967,-68.8916782754277));
#4535=CARTESIAN_POINT('Ctrl Pts',(-101.030778440127,121.913761778509,-68.5765055229452));
#4536=CARTESIAN_POINT('Ctrl Pts',(-100.960164861362,121.882510881795,-68.2634583404383));
#4537=CARTESIAN_POINT('Ctrl Pts',(-100.712810634339,121.813417983957,-67.5935677254039));
#4538=CARTESIAN_POINT('Ctrl Pts',(-100.483220636953,121.771343589081,-67.2056047409378));
#4539=CARTESIAN_POINT('Ctrl Pts',(-99.9029587467504,121.711697111731,-66.5303819021385));
#4540=CARTESIAN_POINT('Ctrl Pts',(-99.5520623213409,121.694880858045,-66.2432484721442));
#4541=CARTESIAN_POINT('Ctrl Pts',(-99.1908428113955,121.694880858045,-66.0346982908408));
#4542=CARTESIAN_POINT('Ctrl Pts',(-98.8578333531796,121.694880858045,-65.8424351904971));
#4543=CARTESIAN_POINT('Ctrl Pts',(-98.4675142149001,121.709425126322,-65.6899158622252));
#4544=CARTESIAN_POINT('Ctrl Pts',(-97.6636618634519,121.766292452039,-65.5478256106297));
#4545=CARTESIAN_POINT('Ctrl Pts',(-97.2499629860219,121.808024204338,-65.5589567845263));
#4546=CARTESIAN_POINT('Ctrl Pts',(-96.532228635356,121.885750778307,-65.7270017969835));
#4547=CARTESIAN_POINT('Ctrl Pts',(-96.1806212553106,121.926229231586,-65.8836810953591));
#4548=CARTESIAN_POINT('Ctrl Pts',(-95.5755231979279,121.983802794611,-66.3313873276683));
#4549=CARTESIAN_POINT('Ctrl Pts',(-95.3217546974658,121.999999999998,-66.6221537056877));
#4550=CARTESIAN_POINT('Ctrl Pts',(-94.9650500672789,121.999999999998,-67.2399842484664));
#4551=CARTESIAN_POINT('Ctrl Pts',(-94.8401232475787,121.983802794611,-67.6051374055565));
#4552=CARTESIAN_POINT('Ctrl Pts',(-94.7903548426391,121.950162492739,-68.0421265757317));
#4553=CARTESIAN_POINT('Ctrl Pts',(-94.7854013049624,121.944988182178,-68.1054231196404));
#4554=CARTESIAN_POINT('Ctrl Pts',(-94.7826830987084,121.93955176967,-68.168721384132));
#4555=CARTESIAN_POINT('Ctrl Pts',(-94.7826830987083,121.93955176967,-68.168721384132));
#4556=CARTESIAN_POINT('Ctrl Pts',(-94.7692793143766,121.912744201006,-68.4808523287743));
#4557=CARTESIAN_POINT('Ctrl Pts',(-94.8123721828179,121.87944427626,-68.7931115535356));
#4558=CARTESIAN_POINT('Ctrl Pts',(-95.0083986686057,121.808024204338,-69.4414600707244));
#4559=CARTESIAN_POINT('Ctrl Pts',(-95.2056082279524,121.766292452039,-69.8052993950442));
#4560=CARTESIAN_POINT('Ctrl Pts',(-95.7305881711883,121.709425126322,-70.4304108264924));
#4561=CARTESIAN_POINT('Ctrl Pts',(-96.0578333531797,121.694880858045,-70.6921774516898));
#4562=CARTESIAN_POINT('Ctrl Pts',(-96.7520623213409,121.694880858045,-71.0929907333369));
#4563=CARTESIAN_POINT('Ctrl Pts',(-97.1761753786965,121.711697111731,-71.2533092368416));
#4564=CARTESIAN_POINT('Ctrl Pts',(-98.0510664554135,121.771343589081,-71.4182193552053));
#4565=CARTESIAN_POINT('Ctrl Pts',(-98.5018472543822,121.813417983957,-71.4230686331636));
#4566=CARTESIAN_POINT('Ctrl Pts',(-99.2682419576485,121.888653805311,-71.2916044625037));
#4567=CARTESIAN_POINT('Ctrl Pts',(-99.6421808158843,121.927100882661,-71.163309142685));
#4568=CARTESIAN_POINT('Ctrl Pts',(-100.289083992022,121.983258351228,-70.7579195346131));
#4569=CARTESIAN_POINT('Ctrl Pts',(-100.561342752554,121.999999999998,-70.4795670133904));
#4570=CARTESIAN_POINT('Ctrl Pts',(-100.92546201219,121.999999999998,-69.8488939556873));
#4571=CARTESIAN_POINT('Ctrl Pts',(-101.03039298651,121.983258351228,-69.4739346920516));
#4572=CARTESIAN_POINT('Ctrl Pts',(-101.046625787479,121.950260836241,-69.0256457187578));
#4573=CARTESIAN_POINT('Ctrl Pts',(-101.046412113711,121.945029125677,-68.9586156139657));
#4574=CARTESIAN_POINT('Ctrl Pts',(-101.043673435707,121.93955176967,-68.8916782754277));
#4575=CARTESIAN_POINT('',(-89.6457108608091,121.928269354306,-62.1822365876521));
#4576=CARTESIAN_POINT('',(-83.8969144629603,121.928269354306,-62.0126448588956));
#4577=CARTESIAN_POINT('Ctrl Pts',(-89.6457108608091,121.928269354306,-62.1822365876521));
#4578=CARTESIAN_POINT('Ctrl Pts',(-89.640048215299,121.903866743648,-61.9118469440624));
#4579=CARTESIAN_POINT('Ctrl Pts',(-89.5938110699338,121.875525701933,-61.6447310127997));
#4580=CARTESIAN_POINT('Ctrl Pts',(-89.4114212651875,121.810267922929,-61.0498367272997));
#4581=CARTESIAN_POINT('Ctrl Pts',(-89.2283577823594,121.76941928365,-60.6962570673076));
#4582=CARTESIAN_POINT('Ctrl Pts',(-88.7408793475757,121.711304602249,-60.0841026261431));
#4583=CARTESIAN_POINT('Ctrl Pts',(-88.4363138250625,121.694880858045,-59.8255680855737));
#4584=CARTESIAN_POINT('Ctrl Pts',(-88.11715467285,121.694880858045,-59.6413014631295));
#4585=CARTESIAN_POINT('Ctrl Pts',(-87.8077521236662,121.694880858045,-59.4626678180703));
#4586=CARTESIAN_POINT('Ctrl Pts',(-87.4431698769551,121.710493799957,-59.3305852473804));
#4587=CARTESIAN_POINT('Ctrl Pts',(-86.6945172380366,121.768237475725,-59.2263000150256));
#4588=CARTESIAN_POINT('Ctrl Pts',(-86.3103592215609,121.809531015002,-59.2542646021946));
#4589=CARTESIAN_POINT('Ctrl Pts',(-85.6299700128694,121.886577617489,-59.4387756069027));
#4590=CARTESIAN_POINT('Ctrl Pts',(-85.2887695763051,121.927161354661,-59.6051048904537));
#4591=CARTESIAN_POINT('Ctrl Pts',(-84.7006180249038,121.984260557561,-60.0622377416933));
#4592=CARTESIAN_POINT('Ctrl Pts',(-84.4534935750556,121.999999999998,-60.35291487129));
#4593=CARTESIAN_POINT('Ctrl Pts',(-84.1015994130934,121.999999999998,-60.9624134386954));
#4594=CARTESIAN_POINT('Ctrl Pts',(-83.9734278594876,121.98426055756,-61.3217680549585));
#4595=CARTESIAN_POINT('Ctrl Pts',(-83.9077720873625,121.947439165029,-61.7976287162892));
#4596=CARTESIAN_POINT('Ctrl Pts',(-83.8992173832946,121.938193561674,-61.9053402793198));
#4597=CARTESIAN_POINT('Ctrl Pts',(-83.8969144629603,121.928269354306,-62.0126448588956));
#4598=CARTESIAN_POINT('Ctrl Pts',(-83.8969144629603,121.928269354306,-62.0126448588956));
#4599=CARTESIAN_POINT('Ctrl Pts',(-83.8912689889189,121.903940742393,-62.2756957380355));
#4600=CARTESIAN_POINT('Ctrl Pts',(-83.9241062924374,121.875500673982,-62.5363189359234));
#4601=CARTESIAN_POINT('Ctrl Pts',(-84.0785731934348,121.809531015002,-63.1198313945313));
#4602=CARTESIAN_POINT('Ctrl Pts',(-84.246434158778,121.768237475725,-63.4665042894511));
#4603=CARTESIAN_POINT('Ctrl Pts',(-84.7110741386961,121.710493799957,-64.0627138771875));
#4604=CARTESIAN_POINT('Ctrl Pts',(-85.0077521236662,121.694880858045,-64.3124100792631));
#4605=CARTESIAN_POINT('Ctrl Pts',(-85.6363138250625,121.694880858045,-64.6753103467665));
#4606=CARTESIAN_POINT('Ctrl Pts',(-86.012494066208,121.711304602249,-64.8098045560952));
#4607=CARTESIAN_POINT('Ctrl Pts',(-86.7863745806878,121.76941928365,-64.9258960438327));
#4608=CARTESIAN_POINT('Ctrl Pts',(-87.1841152899164,121.810267922929,-64.907643840471));
#4609=CARTESIAN_POINT('Ctrl Pts',(-87.8886874328802,121.886091946244,-64.7455648365782));
#4610=CARTESIAN_POINT('Ctrl Pts',(-88.245336954858,121.9263037894,-64.5935914546221));
#4611=CARTESIAN_POINT('Ctrl Pts',(-88.8607180558249,121.983695909948,-64.1544777755007));
#4612=CARTESIAN_POINT('Ctrl Pts',(-89.1191660952628,121.999999999998,-63.866826235406));
#4613=CARTESIAN_POINT('Ctrl Pts',(-89.4775721811683,121.999999999998,-63.2460486848757));
#4614=CARTESIAN_POINT('Ctrl Pts',(-89.5974617026091,121.983695909948,-62.8784003471169));
#4615=CARTESIAN_POINT('Ctrl Pts',(-89.6440171485706,121.946889139357,-62.3958111209995));
#4616=CARTESIAN_POINT('Ctrl Pts',(-89.6479419658163,121.937884080627,-62.2887711900116));
#4617=CARTESIAN_POINT('Ctrl Pts',(-89.6457108608091,121.928269354306,-62.1822365876521));
#4618=CARTESIAN_POINT('',(-75.5607164801933,121.77184403287,-52.8249999999979));
#4619=CARTESIAN_POINT('',(-75.5607164801932,121.77184403287,-58.4249999999981));
#4620=CARTESIAN_POINT('Ctrl Pts',(-75.5607164801933,121.77184403287,-52.8249999999979));
#4621=CARTESIAN_POINT('Ctrl Pts',(-75.31087199813,121.795561855846,-52.8249999999979));
#4622=CARTESIAN_POINT('Ctrl Pts',(-75.0641712044988,121.822609441991,-52.8592756004775));
#4623=CARTESIAN_POINT('Ctrl Pts',(-74.4972946958141,121.886557224277,-53.0111697031877));
#4624=CARTESIAN_POINT('Ctrl Pts',(-74.1537701819123,121.927083062952,-53.1755443283788));
#4625=CARTESIAN_POINT('Ctrl Pts',(-73.561230066802,121.984194331231,-53.6296591429951));
#4626=CARTESIAN_POINT('Ctrl Pts',(-73.3122219315277,121.999999999998,-53.9195067988283));
#4627=CARTESIAN_POINT('Ctrl Pts',(-72.9594687676658,121.999999999998,-54.5304932011677));
#4628=CARTESIAN_POINT('Ctrl Pts',(-72.8329574021241,121.984194331231,-54.8910643999808));
#4629=CARTESIAN_POINT('Ctrl Pts',(-72.7359524939867,121.927083062952,-55.6312765997358));
#4630=CARTESIAN_POINT('Ctrl Pts',(-72.7653621497846,121.886557224277,-56.010964868193));
#4631=CARTESIAN_POINT('Ctrl Pts',(-72.9468930668116,121.810132271938,-56.6884474736823));
#4632=CARTESIAN_POINT('Ctrl Pts',(-73.1112681701126,121.769187929666,-57.0319552746733));
#4633=CARTESIAN_POINT('Ctrl Pts',(-73.5653642866542,121.711112887006,-57.6244722503148));
#4634=CARTESIAN_POINT('Ctrl Pts',(-73.855200110294,121.694880858045,-57.8734811721914));
#4635=CARTESIAN_POINT('Ctrl Pts',(-74.4662328500925,121.694880858045,-58.2262610889977));
#4636=CARTESIAN_POINT('Ctrl Pts',(-74.8267988140265,121.711112887006,-58.3527618142583));
#4637=CARTESIAN_POINT('Ctrl Pts',(-75.3177281966151,121.749631404864,-58.4170976637661));
#4638=CARTESIAN_POINT('Ctrl Pts',(-75.4395919608409,121.760345640413,-58.4249999999981));
#4639=CARTESIAN_POINT('Ctrl Pts',(-75.560716480193,121.77184403287,-58.4249999999981));
#4640=CARTESIAN_POINT('Ctrl Pts',(-75.560716480193,121.77184403287,-58.4249999999981));
#4641=CARTESIAN_POINT('Ctrl Pts',(-75.8105609622564,121.795561855846,-58.4249999999981));
#4642=CARTESIAN_POINT('Ctrl Pts',(-76.0572617558877,121.822609441991,-58.3907243995186));
#4643=CARTESIAN_POINT('Ctrl Pts',(-76.6241382645725,121.886557224277,-58.2388302968083));
#4644=CARTESIAN_POINT('Ctrl Pts',(-76.9676627784743,121.927083062952,-58.0744556716172));
#4645=CARTESIAN_POINT('Ctrl Pts',(-77.5602028935846,121.984194331231,-57.620340857001));
#4646=CARTESIAN_POINT('Ctrl Pts',(-77.8092110288589,121.999999999998,-57.3304932011678));
#4647=CARTESIAN_POINT('Ctrl Pts',(-78.1619641927208,121.999999999998,-56.7195067988283));
#4648=CARTESIAN_POINT('Ctrl Pts',(-78.2884755582626,121.984194331231,-56.3589356000152));
#4649=CARTESIAN_POINT('Ctrl Pts',(-78.3854804663999,121.927083062952,-55.6187234002602));
#4650=CARTESIAN_POINT('Ctrl Pts',(-78.356070810602,121.886557224277,-55.239035131803));
#4651=CARTESIAN_POINT('Ctrl Pts',(-78.174539893575,121.810132271938,-54.5615525263137));
#4652=CARTESIAN_POINT('Ctrl Pts',(-78.010164790274,121.769187929666,-54.2180447253227));
#4653=CARTESIAN_POINT('Ctrl Pts',(-77.5560686737324,121.711112887006,-53.6255277496812));
#4654=CARTESIAN_POINT('Ctrl Pts',(-77.2662328500926,121.694880858045,-53.3765188278046));
#4655=CARTESIAN_POINT('Ctrl Pts',(-76.9607164801934,121.694880858045,-53.2001288694015));
#4656=CARTESIAN_POINT('Ctrl Pts',(-76.6552001102941,121.694880858045,-53.0237389109983));
#4657=CARTESIAN_POINT('Ctrl Pts',(-76.2946341463601,121.711112887006,-52.8972381857377));
#4658=CARTESIAN_POINT('Ctrl Pts',(-75.8037047637714,121.749631404864,-52.8329023362299));
#4659=CARTESIAN_POINT('Ctrl Pts',(-75.6818409995455,121.760345640413,-52.8249999999979));
#4660=CARTESIAN_POINT('Ctrl Pts',(-75.5607164801933,121.77184403287,-52.8249999999979));
#4661=CARTESIAN_POINT('Origin',(-115.614391405224,109.,-78.7499999999976));
#4662=CARTESIAN_POINT('Origin',(-111.692877174869,125.221825406948,-76.4859127034721));
#4663=CARTESIAN_POINT('',(-109.047125863805,127.513113254426,-76.4859127034721));
#4664=CARTESIAN_POINT('Origin',(-111.692877174869,125.221825406948,-76.4859127034721));
#4665=CARTESIAN_POINT('',(-109.576276126018,127.054855684931,-76.4859127034722));
#4666=CARTESIAN_POINT('Origin',(-111.692877174869,125.221825406948,-76.4859127034722));
#4667=CARTESIAN_POINT('Origin',(-111.692877174869,125.221825406948,-76.4859127034721));
#4668=CARTESIAN_POINT('',(-109.047125863805,127.513113254426,-76.4859127034721));
#4669=CARTESIAN_POINT('Origin',(-75.5607164801933,112.,-55.624999999998));
#4670=CARTESIAN_POINT('',(-75.5607164801933,112.,-58.4249999999981));
#4671=CARTESIAN_POINT('Origin',(-84.3932587967998,111.68028146752,-60.7244706841197));
#4672=CARTESIAN_POINT('',(-81.6657313432502,112.313206415782,-60.7244706841197));
#4673=CARTESIAN_POINT('Origin',(-93.3501356426365,112.813466520527,-65.8957259421618));
#4674=CARTESIAN_POINT('',(-90.8457395078369,114.065664587927,-65.8957259421618));
#4675=CARTESIAN_POINT('Origin',(-103.119663075128,115.322330470337,-71.5361652351663));
#4676=CARTESIAN_POINT('',(-101.003062026277,117.155360748319,-71.5361652351663));
#4677=CARTESIAN_POINT('Origin',(-84.2209705180366,98.999999999999,-40.6249999999996));
#4678=CARTESIAN_POINT('',(-86.8190467293899,101.999999999999,-40.1249999999996));
#4679=CARTESIAN_POINT('Origin',(-84.2209705180366,98.999999999999,-40.6249999999996));
#4680=CARTESIAN_POINT('',(-86.4942872029708,101.624999999999,-40.1874999999995));
#4681=CARTESIAN_POINT('Origin',(-84.2209705180366,98.999999999999,-40.6249999999996));
#4682=CARTESIAN_POINT('Origin',(-26.1968246264604,166.000512499998,-141.125768750001));
#4683=CARTESIAN_POINT('',(-28.7949008378137,169.000512499998,-140.625768750001));
#4684=CARTESIAN_POINT('',(-80.5957703324788,98.5672184524782,-46.904030908994));
#4685=CARTESIAN_POINT('',(-80.5957703324788,98.567218452478,-46.9040309089941));
#4686=CARTESIAN_POINT('',(-82.595770332479,105.495421682753,-43.4399292938557));
#4687=CARTESIAN_POINT('Ctrl Pts',(-80.5957703324787,98.5672184524781,-46.9040309089941));
#4688=CARTESIAN_POINT('Ctrl Pts',(-80.1583076046396,98.5672184524781,-46.6514616853158));
#4689=CARTESIAN_POINT('Ctrl Pts',(-79.731847375509,98.6399471087077,-46.316319579711));
#4690=CARTESIAN_POINT('Ctrl Pts',(-79.0280064685973,98.9402745490956,-45.5660699284182));
#4691=CARTESIAN_POINT('Ctrl Pts',(-78.7496249554672,99.168633673537,-45.1522067177974));
#4692=CARTESIAN_POINT('Ctrl Pts',(-78.3748022679429,99.7108672272503,-44.3867423304201));
#4693=CARTESIAN_POINT('Ctrl Pts',(-78.2527827584179,100.061688880156,-43.983215927173));
#4694=CARTESIAN_POINT('Ctrl Pts',(-78.1901153330479,100.862134488935,-43.2736771449321));
#4695=CARTESIAN_POINT('Ctrl Pts',(-78.2490409596484,101.312629171298,-42.9686854143502));
#4696=CARTESIAN_POINT('Ctrl Pts',(-78.5015571253347,102.1873708287,-42.531314585649));
#4697=CARTESIAN_POINT('Ctrl Pts',(-78.7110997683144,102.666877512603,-42.3713056330979));
#4698=CARTESIAN_POINT('Ctrl Pts',(-79.2661565338858,103.572118612493,-42.2280010610046));
#4699=CARTESIAN_POINT('Ctrl Pts',(-79.6121998656049,103.997338243878,-42.2435068221059));
#4700=CARTESIAN_POINT('Ctrl Pts',(-80.340691634629,104.680250326612,-42.3963983912593));
#4701=CARTESIAN_POINT('Ctrl Pts',(-80.7727618736163,104.984284565641,-42.5440649201448));
#4702=CARTESIAN_POINT('Ctrl Pts',(-81.6811020778789,105.3923634715,-42.9401113983139));
#4703=CARTESIAN_POINT('Ctrl Pts',(-82.15830760464,105.495421682753,-43.1873600701774));
#4704=CARTESIAN_POINT('Ctrl Pts',(-82.595770332479,105.495421682753,-43.4399292938557));
#4705=CARTESIAN_POINT('',(-82.595770332479,105.495421682753,-43.4399292938557));
#4706=CARTESIAN_POINT('Origin',(-66.9004624423481,99.0000000000011,-70.6249999999998));
#4707=CARTESIAN_POINT('',(-69.4985386537014,96.000000000001,-70.1249999999998));
#4708=CARTESIAN_POINT('Origin',(-66.9004624423481,99.0000000000011,-70.6249999999998));
#4709=CARTESIAN_POINT('',(-69.1737791272823,96.375000000001,-70.1874999999998));
#4710=CARTESIAN_POINT('Origin',(-66.9004624423481,99.0000000000011,-70.6249999999998));
#4711=CARTESIAN_POINT('Origin',(-124.924608333924,166.000512500002,29.8757687500004));
#4712=CARTESIAN_POINT('',(-127.522684545277,163.000512500001,30.3757687500005));
#4713=CARTESIAN_POINT('',(-68.5256626279059,105.495421682756,-67.8100707061432));
#4714=CARTESIAN_POINT('',(-68.5256626279059,105.495421682756,-67.8100707061433));
#4715=CARTESIAN_POINT('',(-70.5256626279056,98.5672184524799,-64.3459690910059));
#4716=CARTESIAN_POINT('Ctrl Pts',(-68.5256626279059,105.495421682756,-67.8100707061432));
#4717=CARTESIAN_POINT('Ctrl Pts',(-68.0881999000668,105.495421682756,-67.5575014824649));
#4718=CARTESIAN_POINT('Ctrl Pts',(-67.6354735058005,105.392363471503,-67.2678537093952));
#4719=CARTESIAN_POINT('Ctrl Pts',(-66.8383170924954,104.984284565643,-66.6792312563097));
#4720=CARTESIAN_POINT('Ctrl Pts',(-66.4943990076982,104.680250326615,-66.3788807175702));
#4721=CARTESIAN_POINT('Ctrl Pts',(-65.9977451402748,103.99733824388,-65.8244341237244));
#4722=CARTESIAN_POINT('Ctrl Pts',(-65.8112950913965,103.572118612495,-65.5325046881962));
#4723=CARTESIAN_POINT('Ctrl Pts',(-65.657872108522,102.666877512605,-64.9801591426223));
#4724=CARTESIAN_POINT('Ctrl Pts',(-65.6916726047743,102.187370828702,-64.7186854143503));
#4725=CARTESIAN_POINT('Ctrl Pts',(-65.9441887704605,101.3126291713,-64.2813145856493));
#4726=CARTESIAN_POINT('Ctrl Pts',(-66.1788565437883,100.862134488937,-64.0777876307885));
#4727=CARTESIAN_POINT('Ctrl Pts',(-66.8246688668641,100.061688880158,-63.7772898220283));
#4728=CARTESIAN_POINT('Ctrl Pts',(-67.2351427379364,99.7108672272523,-63.6811986154108));
#4729=CARTESIAN_POINT('Ctrl Pts',(-68.0854656868595,99.1686336735389,-63.623072391033));
#4730=CARTESIAN_POINT('Ctrl Pts',(-68.5830724975138,98.9402745490975,-63.6572262480373));
#4731=CARTESIAN_POINT('Ctrl Pts',(-69.5847282081697,98.6399471087095,-63.8916455279991));
#4732=CARTESIAN_POINT('Ctrl Pts',(-70.0881999000665,98.5672184524799,-64.0933998673275));
#4733=CARTESIAN_POINT('Ctrl Pts',(-70.5256626279056,98.5672184524799,-64.3459690910059));
#4734=CARTESIAN_POINT('',(-70.5256626279056,98.5672184524799,-64.3459690910059));
#4735=CARTESIAN_POINT('Origin',(-96.4746890553668,99.4494897427822,-48.5986671816671));
#4736=CARTESIAN_POINT('',(-94.430917460329,100.684620539947,-45.3897032396429));
#4737=CARTESIAN_POINT('Origin',(-96.4746890553668,99.4494897427822,-48.5986671816671));
#4738=CARTESIAN_POINT('',(-94.6863889097089,100.530229190302,-45.7908237323958));
#4739=CARTESIAN_POINT('Origin',(-96.4746890553669,99.4494897427822,-48.598667181667));
#4740=CARTESIAN_POINT('Origin',(41.8109368646032,203.413715679656,-176.687875705469));
#4741=CARTESIAN_POINT('',(43.8547084596409,204.648846476821,-173.478911763445));
#4742=CARTESIAN_POINT('Origin',(-79.9327200516597,99.449489742784,-77.250197953318));
#4743=CARTESIAN_POINT('',(-77.1059069082159,97.3101804481012,-75.3975017575705));
#4744=CARTESIAN_POINT('Origin',(-79.9327200516597,99.449489742784,-77.250197953318));
#4745=CARTESIAN_POINT('',(-77.4592585511463,97.5775941099365,-75.629088782039));
#4746=CARTESIAN_POINT('Origin',(-79.9327200516597,99.4494897427839,-77.250197953318));
#4747=CARTESIAN_POINT('Origin',(-121.718415623925,203.413715679661,106.553271333508));
#4748=CARTESIAN_POINT('',(-118.891602480482,201.274406384978,108.405967529256));
#4749=CARTESIAN_POINT('Origin',(-108.737631016432,99.7320508075681,-56.2438021535162));
#4750=CARTESIAN_POINT('',(-107.276159708174,100.386816955051,-52.5783713592919));
#4751=CARTESIAN_POINT('Origin',(-108.737631016432,99.7320508075681,-56.2438021535162));
#4752=CARTESIAN_POINT('',(-107.458843621706,100.304971186616,-53.03655020857));
#4753=CARTESIAN_POINT('Origin',(-108.737631016432,99.732050807568,-56.2438021535162));
#4754=CARTESIAN_POINT('Origin',(125.171333134686,225.083486900949,-171.899270921774));
#4755=CARTESIAN_POINT('',(126.632804442944,225.738253048432,-168.23384012755));
#4756=CARTESIAN_POINT('Origin',(-92.6850721331748,99.7320508075696,-84.0476497308099));
#4757=CARTESIAN_POINT('',(-89.6744074864335,97.2884302780867,-83.0655005095853));
#4758=CARTESIAN_POINT('Origin',(-92.6850721331748,99.7320508075696,-84.0476497308099));
#4759=CARTESIAN_POINT('',(-90.0507405672762,97.5938828442721,-83.1882691622385));
#4760=CARTESIAN_POINT('Origin',(-92.6850721331748,99.7320508075696,-84.0476497308099));
#4761=CARTESIAN_POINT('Origin',(-75.8911640975186,225.083486900956,176.351189781088));
#4762=CARTESIAN_POINT('',(-72.8804994507773,222.639866371473,177.333339002313));
#4763=CARTESIAN_POINT('Origin',(-121.472809584586,99.8284271247455,-63.7892135623721));
#4764=CARTESIAN_POINT('',(-120.716880638568,99.8284271247455,-59.8612915381242));
#4765=CARTESIAN_POINT('Origin',(-121.472809584586,99.8284271247455,-63.7892135623721));
#4766=CARTESIAN_POINT('',(-120.81137175682,99.8284271247455,-60.3522817911552));
#4767=CARTESIAN_POINT('Origin',(-121.472809584586,99.8284271247455,-63.7892135623721));
#4768=CARTESIAN_POINT('Origin',(201.051502502506,223.968092727195,-125.859046363603));
#4769=CARTESIAN_POINT('',(201.807431448525,223.968092727195,-121.931124339356));
#4770=CARTESIAN_POINT('Origin',(-105.587179379326,99.8284271247468,-91.303932188134));
#4771=CARTESIAN_POINT('',(-102.563463595252,97.2098124419149,-91.303932188134));
#4772=CARTESIAN_POINT('Origin',(-105.587179379326,99.8284271247468,-91.303932188134));
#4773=CARTESIAN_POINT('',(-102.941428068262,97.5371392772689,-91.303932188134));
#4774=CARTESIAN_POINT('Origin',(-105.587179379326,99.8284271247468,-91.303932188134));
#4775=CARTESIAN_POINT('Origin',(1.92092464970915,223.968092727204,219.045231817999));
#4776=CARTESIAN_POINT('',(4.94464043378298,221.349478044372,219.045231817999));
#4777=CARTESIAN_POINT('Origin',(-74.2616783745156,107.500000000001,-57.8749999999998));
#4778=CARTESIAN_POINT('',(-70.018153895972,98.4000000000012,-68.0249999999999));
#4779=CARTESIAN_POINT('',(-76.080331722463,105.400000000001,-57.5249999999998));
#4780=CARTESIAN_POINT('Origin',(-68.1995005480246,100.500000000001,-68.3749999999999));
#4781=CARTESIAN_POINT('Origin',(-76.8597545858689,107.499999999999,-53.3749999999998));
#4782=CARTESIAN_POINT('',(-84.7405857603073,102.599999999999,-42.5249999999996));
#4783=CARTESIAN_POINT('',(-78.6784079338163,109.599999999999,-53.0249999999997));
#4784=CARTESIAN_POINT('Origin',(-82.9219324123599,100.499999999999,-42.8749999999997));
#4785=CARTESIAN_POINT('Origin',(-83.2326628767165,107.659859266241,-62.734681784761));
#4786=CARTESIAN_POINT('',(-78.5362937027295,99.4008619759398,-73.3917489394908));
#4787=CARTESIAN_POINT('',(-81.2538936763059,106.162342759963,-61.4377944477378));
#4788=CARTESIAN_POINT('Origin',(-80.5150629031402,100.898378482218,-74.6886362765139));
#4789=CARTESIAN_POINT('Origin',(-85.5538547168813,107.659859266239,-58.7142595834813));
#4790=CARTESIAN_POINT('',(-93.1168428791077,101.762970040231,-48.1374969637468));
#4791=CARTESIAN_POINT('',(-84.1232146003549,108.524450824255,-56.4679848240644));
#4792=CARTESIAN_POINT('Origin',(-94.5474829956341,100.898378482216,-50.3837717231637));
#4793=CARTESIAN_POINT('Origin',(-91.6988562010068,107.093266739737,-68.7558258325585));
#4794=CARTESIAN_POINT('',(-90.4035687747792,99.3205545426085,-80.661588117438));
#4795=CARTESIAN_POINT('',(-89.5913909482879,105.3827323691,-68.0683213777014));
#4796=CARTESIAN_POINT('Origin',(-92.511034027498,101.031088913246,-81.3490925722951));
#4797=CARTESIAN_POINT('Origin',(-95.0014150842646,107.093266739736,-63.0356260517679));
#4798=CARTESIAN_POINT('',(-105.290562994975,101.489425216483,-54.8765577560743));
#4799=CARTESIAN_POINT('',(-93.9783851684838,107.551603042974,-60.469824495811));
#4800=CARTESIAN_POINT('Origin',(-106.313592910756,101.031088913245,-57.4423593120313));
#4801=CARTESIAN_POINT('Origin',(-100.382013675912,105.838834764833,-76.2779130879201));
#4802=CARTESIAN_POINT('',(-102.552019676931,99.0560570185445,-88.6522817586846));
#4803=CARTESIAN_POINT('',(-98.2654126270599,104.00580448685,-76.2779130879202));
#4804=CARTESIAN_POINT('Origin',(-104.668620725782,100.889087296527,-88.6522817586846));
#4805=CARTESIAN_POINT('Origin',(-105.857312474343,105.838834764831,-66.7944173824152));
#4806=CARTESIAN_POINT('',(-118.187983361742,100.889087296525,-61.5699982312887));
#4807=CARTESIAN_POINT('',(-105.328162212131,105.838834764831,-64.0448719654417));
#4808=CARTESIAN_POINT('Origin',(-118.717133623955,100.889087296525,-64.3195436482622));
#4809=CARTESIAN_POINT('Origin',(-82.9219324123599,100.499999999999,-42.8749999999996));
#4810=CARTESIAN_POINT('',(-85.1952490972941,103.124999999999,-42.4374999999996));
#4811=CARTESIAN_POINT('Origin',(-82.9219324123599,100.499999999999,-42.8749999999996));
#4812=CARTESIAN_POINT('Origin',(-82.9219324123599,100.499999999999,-42.8749999999996));
#4813=CARTESIAN_POINT('',(-85.1952490972941,103.124999999999,-42.4374999999996));
#4814=CARTESIAN_POINT('Origin',(-68.1995005480247,100.500000000001,-68.3749999999998));
#4815=CARTESIAN_POINT('',(-70.4728172329589,97.875000000001,-67.9374999999998));
#4816=CARTESIAN_POINT('Origin',(-68.1995005480247,100.500000000001,-68.3749999999998));
#4817=CARTESIAN_POINT('Origin',(-68.1995005480247,100.500000000001,-68.3749999999998));
#4818=CARTESIAN_POINT('',(-70.4728172329589,97.875000000001,-67.9374999999998));
#4819=CARTESIAN_POINT('Origin',(-94.5474829956341,100.898378482216,-50.3837717231636));
#4820=CARTESIAN_POINT('',(-92.7591828499761,101.979117929735,-47.5759282738925));
#4821=CARTESIAN_POINT('Origin',(-94.5474829956341,100.898378482216,-50.3837717231636));
#4822=CARTESIAN_POINT('Origin',(-94.5474829956341,100.898378482216,-50.3837717231636));
#4823=CARTESIAN_POINT('',(-92.7591828499761,101.979117929735,-47.5759282738925));
#4824=CARTESIAN_POINT('Origin',(-80.5150629031403,100.898378482218,-74.6886362765138));
#4825=CARTESIAN_POINT('',(-78.041601402627,99.0264828493701,-73.0675271052348));
#4826=CARTESIAN_POINT('Origin',(-80.5150629031403,100.898378482218,-74.6886362765138));
#4827=CARTESIAN_POINT('Origin',(-80.5150629031403,100.898378482218,-74.6886362765138));
#4828=CARTESIAN_POINT('',(-78.041601402627,99.0264828493701,-73.0675271052348));
#4829=CARTESIAN_POINT('Origin',(-106.313592910756,101.031088913245,-57.4423593120312));
#4830=CARTESIAN_POINT('',(-105.03480551603,101.604009292292,-54.235107367085));
#4831=CARTESIAN_POINT('Origin',(-106.313592910756,101.031088913245,-57.4423593120312));
#4832=CARTESIAN_POINT('Origin',(-106.313592910756,101.031088913245,-57.4423593120312));
#4833=CARTESIAN_POINT('',(-105.03480551603,101.604009292292,-54.235107367085));
#4834=CARTESIAN_POINT('Origin',(-92.5110340274981,101.031088913246,-81.349092572295));
#4835=CARTESIAN_POINT('',(-89.8767024615995,98.8929209499488,-80.4897120037236));
#4836=CARTESIAN_POINT('Origin',(-92.5110340274981,101.031088913246,-81.349092572295));
#4837=CARTESIAN_POINT('Origin',(-92.5110340274981,101.031088913246,-81.349092572295));
#4838=CARTESIAN_POINT('',(-89.8767024615995,98.8929209499488,-80.4897120037236));
#4839=CARTESIAN_POINT('Origin',(-118.717133623955,100.889087296525,-64.319543648262));
#4840=CARTESIAN_POINT('',(-118.055695796189,100.889087296525,-60.8826118770452));
#4841=CARTESIAN_POINT('Origin',(-118.717133623955,100.889087296525,-64.319543648262));
#4842=CARTESIAN_POINT('Origin',(-118.717133623955,100.889087296525,-64.319543648262));
#4843=CARTESIAN_POINT('',(-118.055695796189,100.889087296525,-60.8826118770452));
#4844=CARTESIAN_POINT('Origin',(-104.668620725782,100.889087296527,-88.6522817586845));
#4845=CARTESIAN_POINT('',(-102.022869414718,98.5977994490487,-88.6522817586845));
#4846=CARTESIAN_POINT('Origin',(-104.668620725782,100.889087296527,-88.6522817586845));
#4847=CARTESIAN_POINT('Origin',(-104.668620725782,100.889087296527,-88.6522817586845));
#4848=CARTESIAN_POINT('',(-102.022869414718,98.5977994490487,-88.6522817586845));
#4849=CARTESIAN_POINT('Origin',(-125.268934230709,90.999,-76.5975199760558));
#4850=CARTESIAN_POINT('',(-122.424179917669,121.863728726179,-74.9551003076436));
#4851=CARTESIAN_POINT('Origin',(-118.577560436093,90.999,-88.1873193607661));
#4852=CARTESIAN_POINT('',(-115.732806123053,121.863728726179,-86.5448996923539));
#4853=CARTESIAN_POINT('Origin',(-115.529994481957,90.999,-74.0824712601139));
#4854=CARTESIAN_POINT('',(-115.529994481957,122.937359864766,-74.0824712601139));
#4855=CARTESIAN_POINT('',(-115.529994481957,122.937359864766,-74.0824712601139));
#4856=CARTESIAN_POINT('',(-115.529994481957,122.937359864766,-74.082471260114));
#4857=CARTESIAN_POINT('Origin',(-111.529994481957,90.999,-81.0106744903897));
#4858=CARTESIAN_POINT('',(-111.529994481957,122.937359864767,-81.0106744903897));
#4859=CARTESIAN_POINT('',(-111.529994481957,122.937359864767,-81.0106744903897));
#4860=CARTESIAN_POINT('',(-111.529994481957,122.937359864767,-81.0106744903897));
#4861=CARTESIAN_POINT('Ctrl Pts',(-111.529994481957,122.930969193824,-81.0106744903897));
#4862=CARTESIAN_POINT('Ctrl Pts',(-111.529994481957,124.224440992555,-81.0106744903897));
#4863=CARTESIAN_POINT('Ctrl Pts',(-111.850631939497,122.930969193824,-81.1957946128129));
#4864=CARTESIAN_POINT('Ctrl Pts',(-111.850631939497,124.224440992555,-81.1957946128129));
#4865=CARTESIAN_POINT('Ctrl Pts',(-112.595893637265,122.930969193824,-81.3855792709696));
#4866=CARTESIAN_POINT('Ctrl Pts',(-112.595893637265,124.224440992555,-81.3855792709696));
#4867=CARTESIAN_POINT('Ctrl Pts',(-113.856111715799,122.930969193824,-81.0858699693662));
#4868=CARTESIAN_POINT('Ctrl Pts',(-113.856111715799,124.224440992555,-81.0858699693662));
#4869=CARTESIAN_POINT('Ctrl Pts',(-115.066649862454,122.930969193824,-80.2473165597762));
#4870=CARTESIAN_POINT('Ctrl Pts',(-115.066649862454,124.224440992555,-80.2473165597762));
#4871=CARTESIAN_POINT('Ctrl Pts',(-116.043255168468,122.930969193824,-78.9976046091529));
#4872=CARTESIAN_POINT('Ctrl Pts',(-116.043255168468,124.224440992555,-78.9976046091529));
#4873=CARTESIAN_POINT('Ctrl Pts',(-116.637234812114,122.930969193824,-77.5269836293621));
#4874=CARTESIAN_POINT('Ctrl Pts',(-116.637234812114,124.224440992555,-77.5269836293621));
#4875=CARTESIAN_POINT('Ctrl Pts',(-116.758174293921,122.930969193824,-76.0593501373141));
#4876=CARTESIAN_POINT('Ctrl Pts',(-116.758174293921,124.224440992555,-76.0593501373141));
#4877=CARTESIAN_POINT('Ctrl Pts',(-116.387621123593,122.930969193824,-74.8181146161938));
#4878=CARTESIAN_POINT('Ctrl Pts',(-116.387621123593,124.224440992555,-74.8181146161938));
#4879=CARTESIAN_POINT('Ctrl Pts',(-115.850631939497,122.930969193824,-74.2675913825374));
#4880=CARTESIAN_POINT('Ctrl Pts',(-115.850631939497,124.224440992555,-74.2675913825374));
#4881=CARTESIAN_POINT('Ctrl Pts',(-115.529994481957,122.930969193824,-74.0824712601142));
#4882=CARTESIAN_POINT('Ctrl Pts',(-115.529994481957,124.224440992555,-74.0824712601142));
#4883=CARTESIAN_POINT('Ctrl Pts',(-111.529994481957,122.937359864767,-81.0106744903897));
#4884=CARTESIAN_POINT('Ctrl Pts',(-111.655985564703,122.937359864767,-81.0834154759286));
#4885=CARTESIAN_POINT('Ctrl Pts',(-111.789124566157,122.941999166342,-81.1417276437762));
#4886=CARTESIAN_POINT('Ctrl Pts',(-112.132055648316,122.963800802529,-81.2508717728567));
#4887=CARTESIAN_POINT('Ctrl Pts',(-112.344262065112,122.985642902608,-81.2836304965519));
#4888=CARTESIAN_POINT('Ctrl Pts',(-112.890185001658,123.055781639719,-81.2942385303482));
#4889=CARTESIAN_POINT('Ctrl Pts',(-113.222304091371,123.111288356191,-81.2310605511146));
#4890=CARTESIAN_POINT('Ctrl Pts',(-114.040071204807,123.254369388729,-80.9469153854904));
#4891=CARTESIAN_POINT('Ctrl Pts',(-114.507617463249,123.341916036999,-80.64733737895));
#4892=CARTESIAN_POINT('Ctrl Pts',(-115.174813131733,123.441390970383,-80.050767705693));
#4893=CARTESIAN_POINT('Ctrl Pts',(-115.415868442681,123.470261290121,-79.7826739036937));
#4894=CARTESIAN_POINT('Ctrl Pts',(-115.755003463233,123.495239476746,-79.3250674771333));
#4895=CARTESIAN_POINT('Ctrl Pts',(-115.872462661464,123.49998997396,-79.1461011463315));
#4896=CARTESIAN_POINT('Ctrl Pts',(-116.085775238015,123.500009989414,-78.7767368883965));
#4897=CARTESIAN_POINT('Ctrl Pts',(-116.182038306449,123.495284034831,-78.5856508621904));
#4898=CARTESIAN_POINT('Ctrl Pts',(-116.408570505306,123.47040914673,-78.0640352851986));
#4899=CARTESIAN_POINT('Ctrl Pts',(-116.52014584973,123.4416707474,-77.7220494143149));
#4900=CARTESIAN_POINT('Ctrl Pts',(-116.700435952419,123.344280060835,-76.8627043141552));
#4901=CARTESIAN_POINT('Ctrl Pts',(-116.72827833538,123.260349185246,-76.3253510567926));
#4902=CARTESIAN_POINT('Ctrl Pts',(-116.580959608512,123.119417363555,-75.4852207472909));
#4903=CARTESIAN_POINT('Ctrl Pts',(-116.473976785389,123.063000944788,-75.16186977102));
#4904=CARTESIAN_POINT('Ctrl Pts',(-116.194331351315,122.989309527258,-74.6783741194887));
#4905=CARTESIAN_POINT('Ctrl Pts',(-116.055391044604,122.965592809847,-74.5005585112936));
#4906=CARTESIAN_POINT('Ctrl Pts',(-115.831958999688,122.946686478982,-74.2944546113625));
#4907=CARTESIAN_POINT('Ctrl Pts',(-115.771332129154,122.942999951482,-74.2445494425702));
#4908=CARTESIAN_POINT('Ctrl Pts',(-115.650653287831,122.938455031077,-74.1565333304243));
#4909=CARTESIAN_POINT('Ctrl Pts',(-115.591330433288,122.937359864766,-74.1178835881261));
#4910=CARTESIAN_POINT('Ctrl Pts',(-115.529994481957,122.937359864766,-74.0824712601142));
#4911=CARTESIAN_POINT('Origin',(-119.078493020361,109.,-80.7499999999988));
#4912=CARTESIAN_POINT('Origin',(-141.995606772677,139.904097174214,-47.6260732918001));
#4913=CARTESIAN_POINT('',(-111.835491639576,108.363035329266,-93.2952463908106));
#4914=CARTESIAN_POINT('Origin',(-145.341293669985,128.314297789504,-41.8311735994448));
#4915=CARTESIAN_POINT('',(-115.181178536884,96.7732359445553,-87.5003466984555));
#4916=CARTESIAN_POINT('Origin',(-134.275197369886,137.573299096998,-41.6148274600336));
#4917=CARTESIAN_POINT('',(-106.49494062967,105.495421682756,-89.7316435813967));
#4918=CARTESIAN_POINT('',(-106.49494062967,105.495421682756,-89.7316435813967));
#4919=CARTESIAN_POINT('',(-106.49494062967,105.495421682756,-89.7316435813966));
#4920=CARTESIAN_POINT('Origin',(-136.275197369886,130.645095866722,-38.1507258448956));
#4921=CARTESIAN_POINT('',(-108.494940629669,98.5672184524796,-86.2675419662591));
#4922=CARTESIAN_POINT('',(-108.494940629669,98.5672184524796,-86.2675419662591));
#4923=CARTESIAN_POINT('',(-108.494940629669,98.5672184524797,-86.2675419662591));
#4924=CARTESIAN_POINT('Ctrl Pts',(-108.497707871361,98.5704137879512,-86.2627489630519));
#4925=CARTESIAN_POINT('Ctrl Pts',(-107.937618152971,97.9236778885854,-87.2328528121005));
#4926=CARTESIAN_POINT('Ctrl Pts',(-108.818345328902,98.5704137879512,-86.4478690854752));
#4927=CARTESIAN_POINT('Ctrl Pts',(-108.258255610512,97.9236778885854,-87.4179729345238));
#4928=CARTESIAN_POINT('Ctrl Pts',(-109.407402641416,98.750783075701,-86.9082076752565));
#4929=CARTESIAN_POINT('Ctrl Pts',(-108.847312923026,98.1040471763352,-87.8783115243051));
#4930=CARTESIAN_POINT('Ctrl Pts',(-110.000372038795,99.5212554870629,-87.7642069906961));
#4931=CARTESIAN_POINT('Ctrl Pts',(-109.440282320405,98.8745195876971,-88.7343108397447));
#4932=CARTESIAN_POINT('Ctrl Pts',(-110.212301964103,100.674348937882,-88.6552937573345));
#4933=CARTESIAN_POINT('Ctrl Pts',(-109.652212245713,100.027613038516,-89.6253976063831));
#4934=CARTESIAN_POINT('Ctrl Pts',(-110.010968557873,102.034515403089,-89.4458315045219));
#4935=CARTESIAN_POINT('Ctrl Pts',(-109.450878839483,101.387779503723,-90.4159353535705));
#4936=CARTESIAN_POINT('Ctrl Pts',(-109.427009489273,103.394681868296,-90.0154602225416));
#4937=CARTESIAN_POINT('Ctrl Pts',(-108.866919770883,102.74794596893,-90.9855640715902));
#4938=CARTESIAN_POINT('Ctrl Pts',(-108.549340749734,104.547775319115,-90.2774669067221));
#4939=CARTESIAN_POINT('Ctrl Pts',(-107.989251031344,103.901039419749,-91.2475707557707));
#4940=CARTESIAN_POINT('Ctrl Pts',(-107.511538898252,105.318247730477,-90.1919400026446));
#4941=CARTESIAN_POINT('Ctrl Pts',(-106.951449179862,104.671511831111,-91.1620438516932));
#4942=CARTESIAN_POINT('Ctrl Pts',(-106.818345328902,105.498617018227,-89.9119707006131));
#4943=CARTESIAN_POINT('Ctrl Pts',(-106.258255610512,104.851881118861,-90.8820745496617));
#4944=CARTESIAN_POINT('Ctrl Pts',(-106.497707871361,105.498617018227,-89.7268505781898));
#4945=CARTESIAN_POINT('Ctrl Pts',(-105.937618152971,104.851881118861,-90.6969544272384));
#4946=CARTESIAN_POINT('Ctrl Pts',(-108.494940629669,98.5672184524797,-86.2675419662592));
#4947=CARTESIAN_POINT('Ctrl Pts',(-108.620931712415,98.5672184524797,-86.3402829517981));
#4948=CARTESIAN_POINT('Ctrl Pts',(-108.740009575843,98.5788155545531,-86.4229497251191));
#4949=CARTESIAN_POINT('Ctrl Pts',(-109.015792308145,98.634550154098,-86.6483982077968));
#4950=CARTESIAN_POINT('Ctrl Pts',(-109.160240827059,98.6909481351825,-86.7985170532378));
#4951=CARTESIAN_POINT('Ctrl Pts',(-109.477961818401,98.884314307059,-87.2043824505149));
#4952=CARTESIAN_POINT('Ctrl Pts',(-109.620465834967,99.047756217635,-87.4696274118531));
#4953=CARTESIAN_POINT('Ctrl Pts',(-109.88505667753,99.5434281228911,-88.1436116529208));
#4954=CARTESIAN_POINT('Ctrl Pts',(-109.944782655288,99.9267917722889,-88.5503990928816));
#4955=CARTESIAN_POINT('Ctrl Pts',(-109.931222669289,100.613385759641,-89.132932800729));
#4956=CARTESIAN_POINT('Ctrl Pts',(-109.895248991132,100.904400962771,-89.3446672830305));
#4957=CARTESIAN_POINT('Ctrl Pts',(-109.799168414145,101.381966460934,-89.6408763836526));
#4958=CARTESIAN_POINT('Ctrl Pts',(-109.754281345734,101.564677285217,-89.7431020350957));
#4959=CARTESIAN_POINT('Ctrl Pts',(-109.647683916166,101.93405752606,-89.9278381616077));
#4960=CARTESIAN_POINT('Ctrl Pts',(-109.585780717548,102.121418154361,-90.0107041459795));
#4961=CARTESIAN_POINT('Ctrl Pts',(-109.399335228826,102.623158600648,-90.2043869062662));
#4962=CARTESIAN_POINT('Ctrl Pts',(-109.259387572093,102.942330744829,-90.2980516526588));
#4963=CARTESIAN_POINT('Ctrl Pts',(-108.856079275086,103.713602817721,-90.4495286319902));
#4964=CARTESIAN_POINT('Ctrl Pts',(-108.560802720886,104.170639304011,-90.4718337906789));
#4965=CARTESIAN_POINT('Ctrl Pts',(-107.984073142598,104.807412067022,-90.3754648931577));
#4966=CARTESIAN_POINT('Ctrl Pts',(-107.731615284225,105.031808587313,-90.3040840691712));
#4967=CARTESIAN_POINT('Ctrl Pts',(-107.274706570105,105.310186009746,-90.1276174249943));
#4968=CARTESIAN_POINT('Ctrl Pts',(-107.082643892882,105.395243156987,-90.0418124615454));
#4969=CARTESIAN_POINT('Ctrl Pts',(-106.81731713635,105.462525333909,-89.9082723306999));
#4970=CARTESIAN_POINT('Ctrl Pts',(-106.748607297535,105.475545269237,-89.8723672736483));
#4971=CARTESIAN_POINT('Ctrl Pts',(-106.617982888177,105.491574342406,-89.8015773906488));
#4972=CARTESIAN_POINT('Ctrl Pts',(-106.556276581001,105.495421682755,-89.7670559094086));
#4973=CARTESIAN_POINT('Ctrl Pts',(-106.49494062967,105.495421682755,-89.7316435813966));
#4974=CARTESIAN_POINT('Origin',(-119.078493020361,109.,-80.7499999999988));
#4975=CARTESIAN_POINT('Origin',(-98.8802009968175,127.881285087611,-122.304146684539));
#4976=CARTESIAN_POINT('',(-122.975807503838,96.7732359445554,-73.9996533015419));
#4977=CARTESIAN_POINT('Origin',(-102.225887894125,139.471084472322,-116.509246992184));
#4978=CARTESIAN_POINT('',(-126.321494401146,108.363035329266,-68.2047536091869));
#4979=CARTESIAN_POINT('Origin',(-91.1597915940262,130.212083164828,-116.292900852773));
#4980=CARTESIAN_POINT('',(-118.565048334243,98.5672184524784,-68.8256037842474));
#4981=CARTESIAN_POINT('',(-118.565048334243,98.5672184524783,-68.8256037842474));
#4982=CARTESIAN_POINT('',(-118.565048334243,98.5672184524784,-68.8256037842474));
#4983=CARTESIAN_POINT('Origin',(-93.159791594026,137.140286395103,-112.828799237635));
#4984=CARTESIAN_POINT('',(-120.565048334243,105.495421682754,-65.3615021691091));
#4985=CARTESIAN_POINT('',(-120.565048334243,105.495421682754,-65.3615021691091));
#4986=CARTESIAN_POINT('',(-120.565048334243,105.495421682754,-65.3615021691091));
#4987=CARTESIAN_POINT('Ctrl Pts',(-120.562281092551,105.498617018225,-65.3662951723163));
#4988=CARTESIAN_POINT('Ctrl Pts',(-121.122370810941,104.85188111886,-64.3961913232677));
#4989=CARTESIAN_POINT('Ctrl Pts',(-120.882918550091,105.498617018225,-65.5514152947396));
#4990=CARTESIAN_POINT('Ctrl Pts',(-121.443008268481,104.85188111886,-64.581311445691));
#4991=CARTESIAN_POINT('Ctrl Pts',(-121.471975862605,105.318247730476,-66.0117538845209));
#4992=CARTESIAN_POINT('Ctrl Pts',(-122.032065580995,104.67151183111,-65.0416500354723));
#4993=CARTESIAN_POINT('Ctrl Pts',(-122.064945259985,104.547775319114,-66.8677531999604));
#4994=CARTESIAN_POINT('Ctrl Pts',(-122.625034978375,103.901039419748,-65.8976493509118));
#4995=CARTESIAN_POINT('Ctrl Pts',(-122.276875185293,103.394681868295,-67.7588399665989));
#4996=CARTESIAN_POINT('Ctrl Pts',(-122.836964903683,102.747945968929,-66.7887361175503));
#4997=CARTESIAN_POINT('Ctrl Pts',(-122.075541779062,102.034515403088,-68.5493777137862));
#4998=CARTESIAN_POINT('Ctrl Pts',(-122.635631497452,101.387779503722,-67.5792738647376));
#4999=CARTESIAN_POINT('Ctrl Pts',(-121.491582710463,100.674348937881,-69.1190064318059));
#5000=CARTESIAN_POINT('Ctrl Pts',(-122.051672428853,100.027613038515,-68.1489025827573));
#5001=CARTESIAN_POINT('Ctrl Pts',(-120.613913970924,99.5212554870615,-69.3810131159864));
#5002=CARTESIAN_POINT('Ctrl Pts',(-121.174003689314,98.8745195876958,-68.4109092669378));
#5003=CARTESIAN_POINT('Ctrl Pts',(-119.576112119442,98.7507830756997,-69.2954862119089));
#5004=CARTESIAN_POINT('Ctrl Pts',(-120.136201837832,98.104047176334,-68.3253823628603));
#5005=CARTESIAN_POINT('Ctrl Pts',(-118.882918550091,98.5704137879498,-69.0155169098773));
#5006=CARTESIAN_POINT('Ctrl Pts',(-119.443008268481,97.9236778885841,-68.0454130608287));
#5007=CARTESIAN_POINT('Ctrl Pts',(-118.562281092551,98.5704137879498,-68.8303967874541));
#5008=CARTESIAN_POINT('Ctrl Pts',(-119.122370810941,97.9236778885841,-67.8602929384055));
#5009=CARTESIAN_POINT('Ctrl Pts',(-120.565048334243,105.495421682754,-65.3615021691091));
#5010=CARTESIAN_POINT('Ctrl Pts',(-120.691039416989,105.495421682754,-65.4342431546481));
#5011=CARTESIAN_POINT('Ctrl Pts',(-120.814135033437,105.479185279105,-65.509950975606));
#5012=CARTESIAN_POINT('Ctrl Pts',(-121.108798536521,105.401649043373,-65.7026970040038));
#5013=CARTESIAN_POINT('Ctrl Pts',(-121.272162868975,105.32340896221,-65.8200526993256));
#5014=CARTESIAN_POINT('Ctrl Pts',(-121.650625788444,105.059904053223,-66.1207099909364));
#5015=CARTESIAN_POINT('Ctrl Pts',(-121.841200031555,104.840955426175,-66.3026948775666));
#5016=CARTESIAN_POINT('Ctrl Pts',(-122.229702683097,104.20220248838,-66.7620575698267));
#5017=CARTESIAN_POINT('Ctrl Pts',(-122.365246282272,103.731292190713,-67.0375250373832));
#5018=CARTESIAN_POINT('Ctrl Pts',(-122.437834115624,102.945223269976,-67.4708463451536));
#5019=CARTESIAN_POINT('Ctrl Pts',(-122.426862867774,102.625337747109,-67.6392753478494));
#5020=CARTESIAN_POINT('Ctrl Pts',(-122.352414034946,102.122794062321,-67.8980171685339));
#5021=CARTESIAN_POINT('Ctrl Pts',(-122.311641017802,101.935332740824,-67.9931170741559));
#5022=CARTESIAN_POINT('Ctrl Pts',(-122.205060922126,101.565932484526,-68.1778231774862));
#5023=CARTESIAN_POINT('Ctrl Pts',(-122.139064926783,101.383297810808,-68.2677780937319));
#5024=CARTESIAN_POINT('Ctrl Pts',(-121.931077153049,100.906432252622,-68.4987731861706));
#5025=CARTESIAN_POINT('Ctrl Pts',(-121.766241312432,100.615998507772,-68.6355455315589));
#5026=CARTESIAN_POINT('Ctrl Pts',(-121.278590206767,99.9421171214444,-68.9331085407376));
#5027=CARTESIAN_POINT('Ctrl Pts',(-120.910627382145,99.5690115107432,-69.0813100128094));
#5028=CARTESIAN_POINT('Ctrl Pts',(-120.211847266071,99.0731705694225,-69.1963388478251));
#5029=CARTESIAN_POINT('Ctrl Pts',(-119.910531355856,98.9051904678996,-69.2095826519892));
#5030=CARTESIAN_POINT('Ctrl Pts',(-119.389804002114,98.7005044629965,-69.1436531341076));
#5031=CARTESIAN_POINT('Ctrl Pts',(-119.177202045119,98.6391640331656,-69.0934232467741));
#5032=CARTESIAN_POINT('Ctrl Pts',(-118.895501925765,98.5907881871084,-68.988242612226));
#5033=CARTESIAN_POINT('Ctrl Pts',(-118.823599460482,98.5814547792815,-68.9578673464248));
#5034=CARTESIAN_POINT('Ctrl Pts',(-118.689039034596,98.5699706265173,-68.8938948440334));
#5035=CARTESIAN_POINT('Ctrl Pts',(-118.626384285574,98.5672184524785,-68.8610161122592));
#5036=CARTESIAN_POINT('Ctrl Pts',(-118.565048334243,98.5672184524785,-68.8256037842472));
#5037=CARTESIAN_POINT('Origin',(-119.078493020361,109.,-80.7499999999988));
#5038=CARTESIAN_POINT('Origin',(-69.3034604663987,124.991664350565,-51.4350212868557));
#5039=CARTESIAN_POINT('',(-67.366968793295,124.991664350565,-50.3169872981059));
#5040=CARTESIAN_POINT('Origin',(-68.8034604663987,123.191664350565,-52.3010466906402));
#5041=CARTESIAN_POINT('',(-66.866968793295,124.991664350565,-51.1830127018903));
#5042=CARTESIAN_POINT('Origin',(-69.3034604663987,124.991664350565,-51.4350212868557));
#5043=CARTESIAN_POINT('Origin',(-76.346812504256,100.571155122824,-40.3758635351318));
#5044=CARTESIAN_POINT('',(-73.9165625814855,100.571155122824,-38.9727580880221));
#5045=CARTESIAN_POINT('Origin',(-75.81738964085,102.337180526609,-41.2928508332395));
#5046=CARTESIAN_POINT('',(-74.1665625814855,101.437180526609,-38.5397453861299));
#5047=CARTESIAN_POINT('Origin',(-76.346812504256,100.571155122824,-40.3758635351318));
#5048=CARTESIAN_POINT('Origin',(-62.497624927873,101.437180526611,-64.3633600609793));
#5049=CARTESIAN_POINT('',(-60.0673750051025,101.437180526611,-62.9602546138697));
#5050=CARTESIAN_POINT('Origin',(-63.527047791279,101.471155122826,-62.580347359087));
#5051=CARTESIAN_POINT('',(-60.3173750051025,100.571155122826,-62.5272419119774));
#5052=CARTESIAN_POINT('Origin',(-62.497624927873,101.437180526611,-64.3633600609793));
#5171=UNCERTAINTY_MEASURE_WITH_UNIT(LENGTH_MEASURE(0.01),#5184,
'DISTANCE_ACCURACY_VALUE',
'Maximum model space distance between geometric entities at asserted c
onnectivities');
#5176=UNCERTAINTY_MEASURE_WITH_UNIT(LENGTH_MEASURE(0.01),#5184,
'DISTANCE_ACCURACY_VALUE',
'Maximum model space distance between geometric entities at asserted c
onnectivities');
#5178=(
GEOMETRIC_REPRESENTATION_CONTEXT(3)
GLOBAL_UNCERTAINTY_ASSIGNED_CONTEXT((#5171))
GLOBAL_UNIT_ASSIGNED_CONTEXT((#5184,#5186,#5187))
REPRESENTATION_CONTEXT('','3D')
);
#5183=(
GEOMETRIC_REPRESENTATION_CONTEXT(3)
GLOBAL_UNCERTAINTY_ASSIGNED_CONTEXT((#5176))
GLOBAL_UNIT_ASSIGNED_CONTEXT((#5184,#5186,#5187))
REPRESENTATION_CONTEXT('','3D')
);
#5184=(
LENGTH_UNIT()
NAMED_UNIT(*)
SI_UNIT(.MILLI.,.METRE.)
);
#5186=(
NAMED_UNIT(*)
PLANE_ANGLE_UNIT()
SI_UNIT($,.RADIAN.)
);
#5187=(
NAMED_UNIT(*)
SI_UNIT($,.STERADIAN.)
SOLID_ANGLE_UNIT()
);
#5189=SHAPE_DEFINITION_REPRESENTATION(#5195,#5214);
#5195=PRODUCT_DEFINITION_SHAPE('',$,#5221);
#5214=SHAPE_REPRESENTATION('',(#2425),#5178);
#5219=PRODUCT_DEFINITION_CONTEXT('part definition',#5239,'design');
#5221=PRODUCT_DEFINITION('Sprinkler','Sprinkler',#5227,#5219);
#5227=PRODUCT_DEFINITION_FORMATION('',$,#5242);
#5239=APPLICATION_CONTEXT(
'Core Data for Automotive Mechanical Design Process');
#5240=PRODUCT_CONTEXT('part definition',#5239,'mechanical');
#5242=PRODUCT('Sprinkler','Sprinkler',$,(#5240));
#5247=PRESENTATION_STYLE_ASSIGNMENT((#5248));
#5248=SURFACE_STYLE_USAGE(.BOTH.,#5249);
#5249=SURFACE_SIDE_STYLE('',(#5250));
#5250=SURFACE_STYLE_FILL_AREA(#5251);
#5251=FILL_AREA_STYLE('Steel - Satin',(#5252));
#5252=FILL_AREA_STYLE_COLOUR('Steel - Satin',#5253);
#5253=COLOUR_RGB('Steel - Satin',0.627450980392157,0.627450980392157,0.627450980392157);
ENDSEC;
END-ISO-10303-21;
